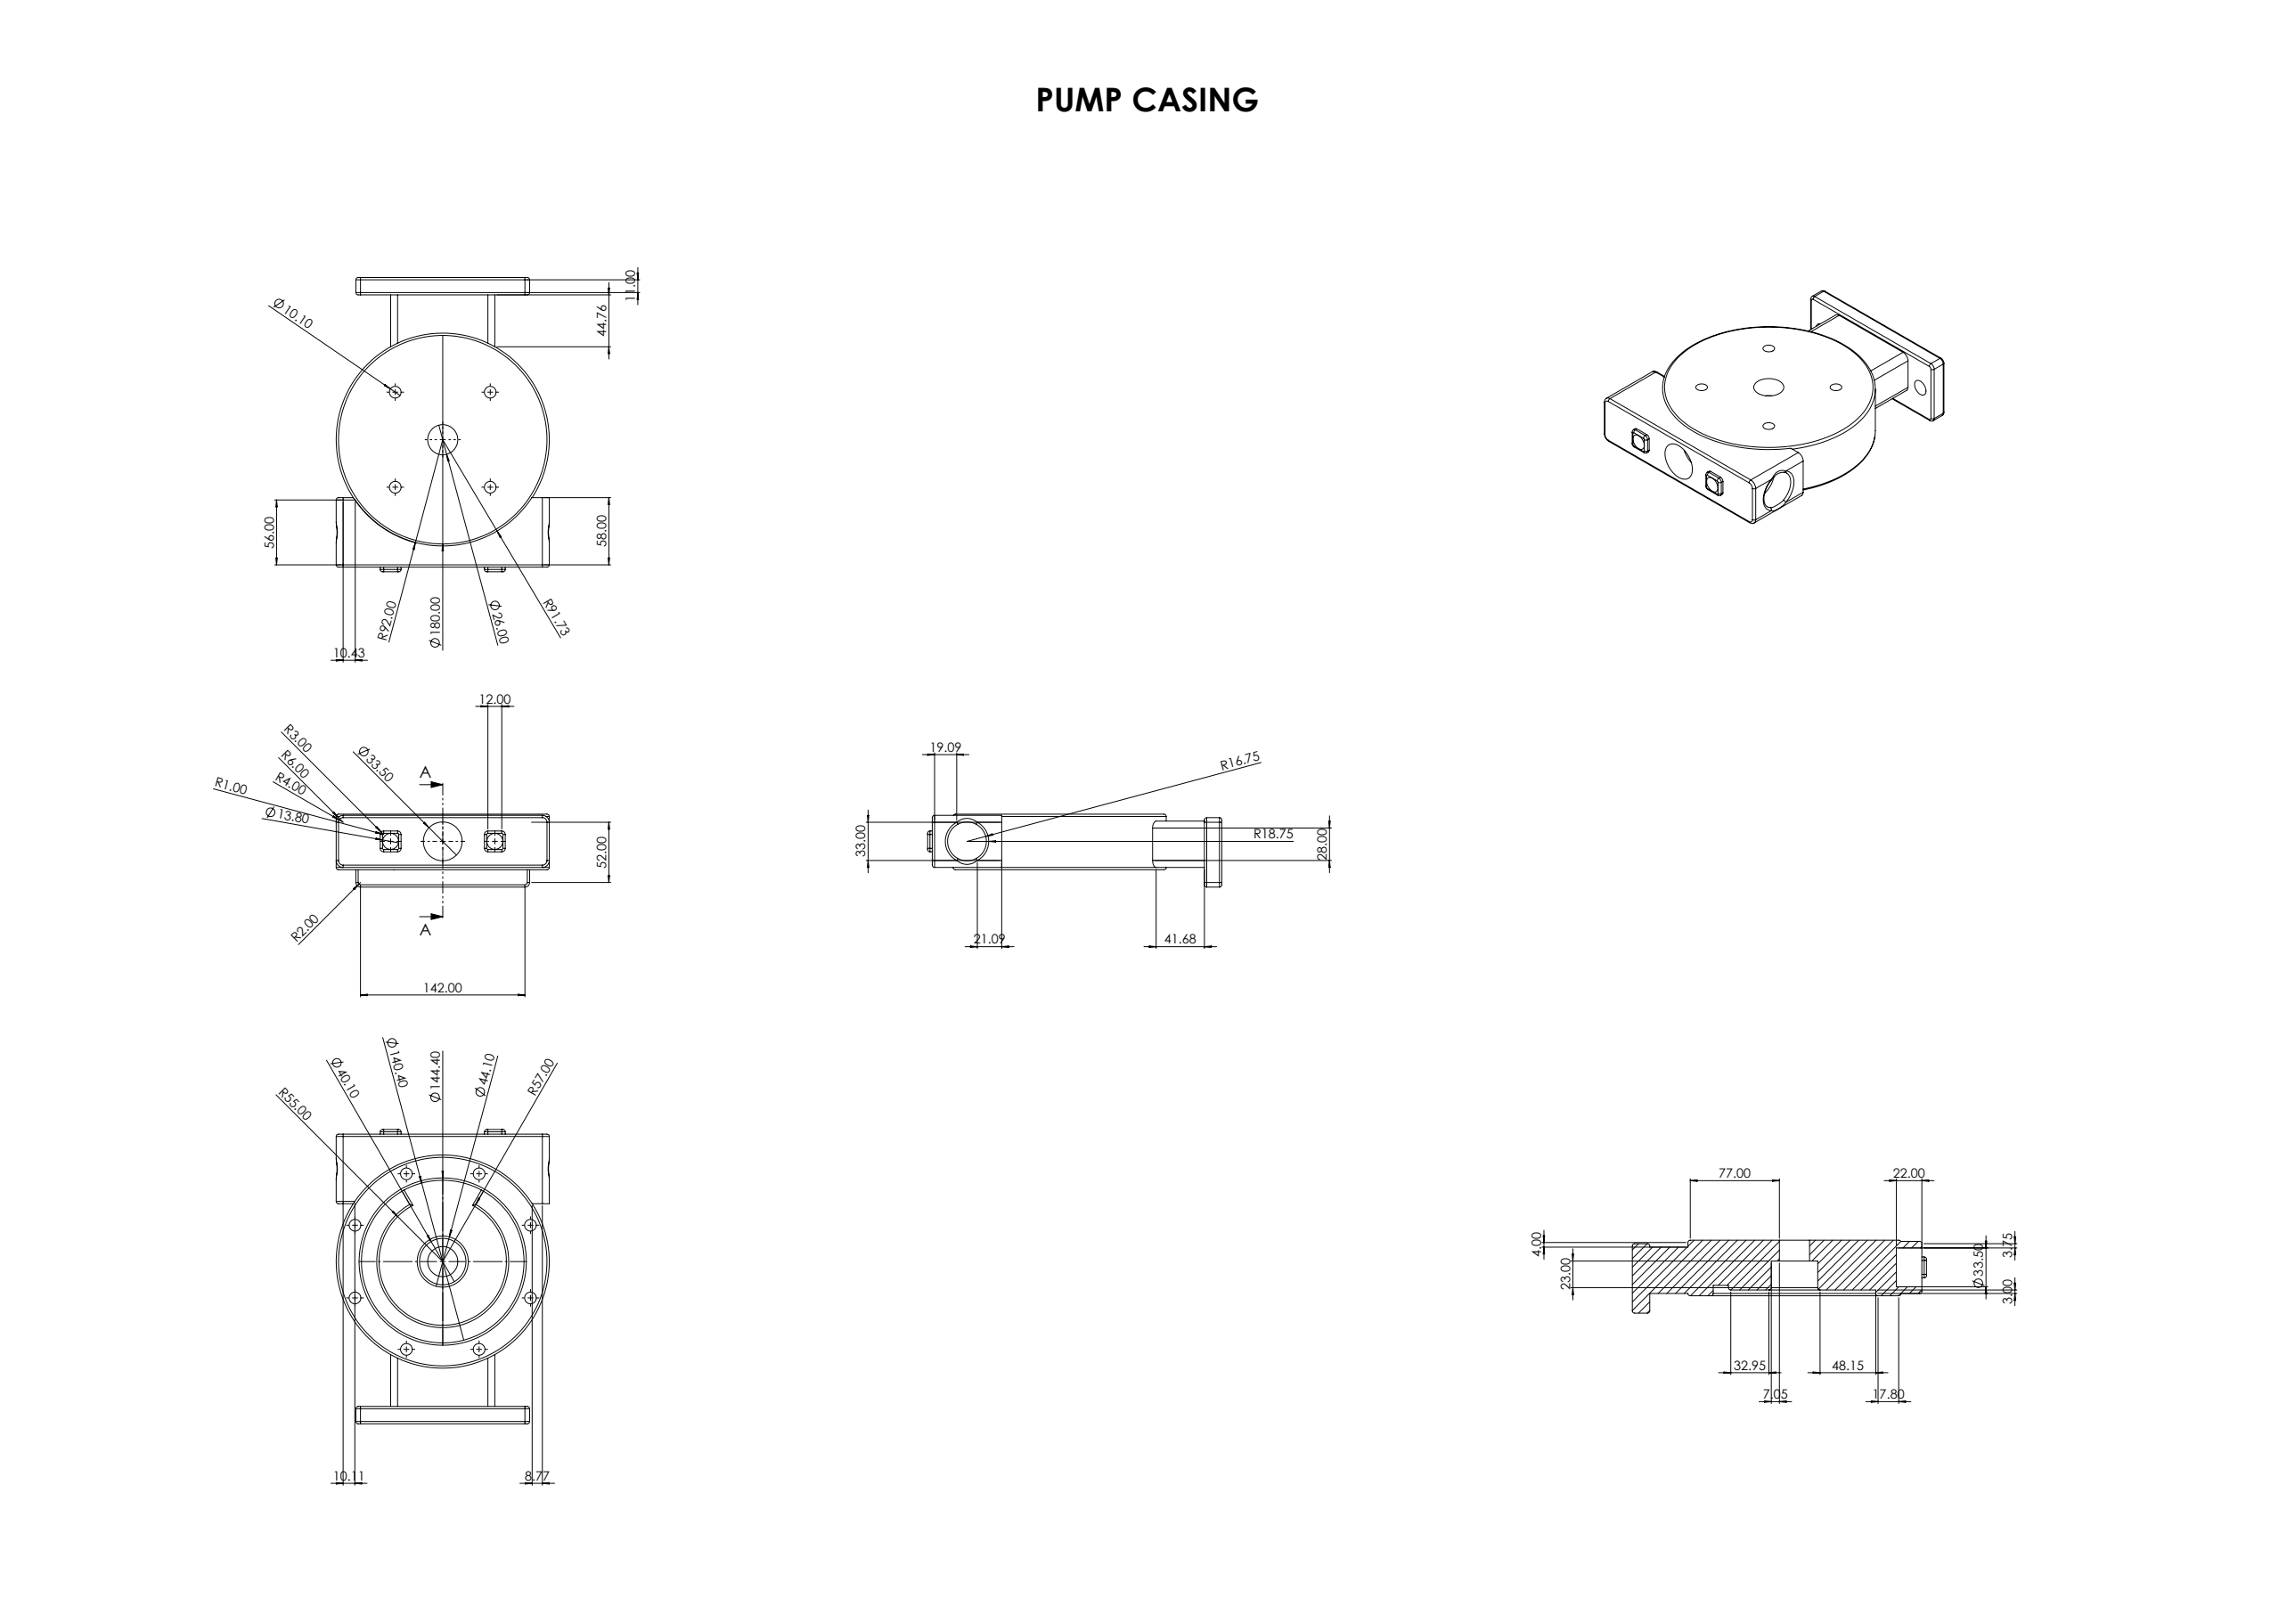
ISO-10303-21;
HEADER;
/* Generated by software containing ST-Developer
 * from STEP Tools, Inc. (www.steptools.com) 
 */

FILE_DESCRIPTION(
/* description */ (''),
/* implementation_level */ '2;1');

FILE_NAME(
/* name */ '01_Pump_Casing.step',
/* time_stamp */ '2026-10-26T04:15:57-07:00',
/* author */ (''),
/* organization */ (''),
/* preprocessor_version */ 'ST-DEVELOPER v20.2',
/* originating_system */ 'Autodesk Translation Framework v15.15.0.0',
/* authorisation */ '');

FILE_SCHEMA (('AUTOMOTIVE_DESIGN { 1 0 10303 214 3 1 1 }'));
ENDSEC;

DATA;
#10=MECHANICAL_DESIGN_GEOMETRIC_PRESENTATION_REPRESENTATION('',(#452),#55737);
#412=SHAPE_REPRESENTATION_RELATIONSHIP('SRR','None',#55821,#432);
#432=ADVANCED_BREP_SHAPE_REPRESENTATION('',(#472),#55717);
#452=STYLED_ITEM('',(#56005),#472);
#472=MANIFOLD_SOLID_BREP('Body1',#27221);
#492=B_SPLINE_SURFACE_WITH_KNOTS('',3,3,((#38041,#38042,#38043,#38044,#38045,
#38046,#38047,#38048),(#38049,#38050,#38051,#38052,#38053,#38054,#38055,
#38056),(#38057,#38058,#38059,#38060,#38061,#38062,#38063,#38064),(#38065,
#38066,#38067,#38068,#38069,#38070,#38071,#38072),(#38073,#38074,#38075,
#38076,#38077,#38078,#38079,#38080),(#38081,#38082,#38083,#38084,#38085,
#38086,#38087,#38088)),.UNSPECIFIED.,.F.,.F.,.F.,(4,1,1,4),(4,1,1,1,1,4),
(0.,0.285714285714286,0.571428571428571,1.),(0.,0.532095912060411,0.798143868090616,
1.06419182412082,1.59628773618123,1.86233569221144),.UNSPECIFIED.);
#493=B_SPLINE_SURFACE_WITH_KNOTS('',3,3,((#38114,#38115,#38116,#38117,#38118,
#38119,#38120,#38121),(#38122,#38123,#38124,#38125,#38126,#38127,#38128,
#38129),(#38130,#38131,#38132,#38133,#38134,#38135,#38136,#38137),(#38138,
#38139,#38140,#38141,#38142,#38143,#38144,#38145),(#38146,#38147,#38148,
#38149,#38150,#38151,#38152,#38153),(#38154,#38155,#38156,#38157,#38158,
#38159,#38160,#38161)),.UNSPECIFIED.,.F.,.F.,.F.,(4,1,1,4),(4,1,1,1,1,4),
(0.,0.285714285714286,0.571428571428571,1.),(8.87358627225765E-17,0.532095912059373,
0.798143868089059,1.06419182411875,1.33023978014843,1.8623356922078),
 .UNSPECIFIED.);
#494=B_SPLINE_SURFACE_WITH_KNOTS('',3,3,((#38313,#38314,#38315,#38316,#38317,
#38318,#38319,#38320,#38321),(#38322,#38323,#38324,#38325,#38326,#38327,
#38328,#38329,#38330),(#38331,#38332,#38333,#38334,#38335,#38336,#38337,
#38338,#38339),(#38340,#38341,#38342,#38343,#38344,#38345,#38346,#38347,
#38348),(#38349,#38350,#38351,#38352,#38353,#38354,#38355,#38356,#38357),
(#38358,#38359,#38360,#38361,#38362,#38363,#38364,#38365,#38366)),
 .UNSPECIFIED.,.F.,.F.,.F.,(4,1,1,4),(4,1,1,1,1,1,4),(0.,0.285714285714286,
0.571428571428571,1.),(0.,0.266047956030205,0.798143868090615,1.06419182412082,
1.33023978015103,1.46326375816613,1.86233569221144),.UNSPECIFIED.);
#495=B_SPLINE_SURFACE_WITH_KNOTS('',3,3,((#38384,#38385,#38386,#38387,#38388,
#38389,#38390,#38391),(#38392,#38393,#38394,#38395,#38396,#38397,#38398,
#38399),(#38400,#38401,#38402,#38403,#38404,#38405,#38406,#38407),(#38408,
#38409,#38410,#38411,#38412,#38413,#38414,#38415),(#38416,#38417,#38418,
#38419,#38420,#38421,#38422,#38423),(#38424,#38425,#38426,#38427,#38428,
#38429,#38430,#38431)),.UNSPECIFIED.,.F.,.F.,.F.,(4,1,1,4),(4,1,1,1,1,4),
(0.,0.285714285714286,0.571428571428571,1.),(2.59005157847017E-16,0.532095912059373,
0.79814386808906,1.06419182411875,1.59628773617812,1.86233569220781),
 .UNSPECIFIED.);
#584=(
BOUNDED_SURFACE()
B_SPLINE_SURFACE(2,2,((#37536,#37537,#37538),(#37539,#37540,#37541),(#37542,
#37543,#37544)),.UNSPECIFIED.,.F.,.F.,.F.)
B_SPLINE_SURFACE_WITH_KNOTS((3,3),(3,3),(-1.5707963267949,0.),(-3.14159265358979,
-1.5707963267949),.UNSPECIFIED.)
GEOMETRIC_REPRESENTATION_ITEM()
RATIONAL_B_SPLINE_SURFACE(((1.,0.707106781186549,1.),(0.707106781186545,
0.499999999999999,0.707106781186545),(1.,0.707106781186549,1.)))
REPRESENTATION_ITEM('')
SURFACE()
);
#585=(
BOUNDED_SURFACE()
B_SPLINE_SURFACE(2,2,((#37556,#37557,#37558),(#37559,#37560,#37561),(#37562,
#37563,#37564)),.UNSPECIFIED.,.F.,.F.,.F.)
B_SPLINE_SURFACE_WITH_KNOTS((3,3),(3,3),(-1.5707963267949,0.),(-1.5707963267949,
-4.44089209850058E-15),.UNSPECIFIED.)
GEOMETRIC_REPRESENTATION_ITEM()
RATIONAL_B_SPLINE_SURFACE(((1.,0.707106781186549,1.),(0.707106781186545,
0.499999999999999,0.707106781186545),(1.,0.707106781186549,1.)))
REPRESENTATION_ITEM('')
SURFACE()
);
#586=(
BOUNDED_SURFACE()
B_SPLINE_SURFACE(2,2,((#37576,#37577,#37578),(#37579,#37580,#37581),(#37582,
#37583,#37584)),.UNSPECIFIED.,.F.,.F.,.F.)
B_SPLINE_SURFACE_WITH_KNOTS((3,3),(3,3),(-1.5707963267949,0.),(4.4408920985006E-15,
1.57079632679489),.UNSPECIFIED.)
GEOMETRIC_REPRESENTATION_ITEM()
RATIONAL_B_SPLINE_SURFACE(((1.,0.70710678118655,1.),(0.707106781186545,
0.5,0.707106781186545),(1.,0.70710678118655,1.)))
REPRESENTATION_ITEM('')
SURFACE()
);
#587=(
BOUNDED_SURFACE()
B_SPLINE_SURFACE(2,2,((#37596,#37597,#37598),(#37599,#37600,#37601),(#37602,
#37603,#37604)),.UNSPECIFIED.,.F.,.F.,.F.)
B_SPLINE_SURFACE_WITH_KNOTS((3,3),(3,3),(-1.5707963267949,0.),(1.5707963267949,
3.14159265358979),.UNSPECIFIED.)
GEOMETRIC_REPRESENTATION_ITEM()
RATIONAL_B_SPLINE_SURFACE(((1.,0.707106781186549,1.),(0.707106781186545,
0.499999999999999,0.707106781186545),(1.,0.707106781186549,1.)))
REPRESENTATION_ITEM('')
SURFACE()
);
#588=(
BOUNDED_SURFACE()
B_SPLINE_SURFACE(2,2,((#37639,#37640,#37641),(#37642,#37643,#37644),(#37645,
#37646,#37647)),.UNSPECIFIED.,.F.,.F.,.F.)
B_SPLINE_SURFACE_WITH_KNOTS((3,3),(3,3),(0.,1.5707963267949),(-1.5707963267949,
-4.44089209850058E-15),.UNSPECIFIED.)
GEOMETRIC_REPRESENTATION_ITEM()
RATIONAL_B_SPLINE_SURFACE(((1.,0.707106781186549,1.),(0.707106781186545,
0.499999999999999,0.707106781186545),(1.,0.707106781186549,1.)))
REPRESENTATION_ITEM('')
SURFACE()
);
#589=(
BOUNDED_SURFACE()
B_SPLINE_SURFACE(2,2,((#37658,#37659,#37660),(#37661,#37662,#37663),(#37664,
#37665,#37666)),.UNSPECIFIED.,.F.,.F.,.F.)
B_SPLINE_SURFACE_WITH_KNOTS((3,3),(3,3),(0.,1.5707963267949),(4.4408920985006E-15,
1.57079632679489),.UNSPECIFIED.)
GEOMETRIC_REPRESENTATION_ITEM()
RATIONAL_B_SPLINE_SURFACE(((1.,0.70710678118655,1.),(0.707106781186545,
0.5,0.707106781186545),(1.,0.70710678118655,1.)))
REPRESENTATION_ITEM('')
SURFACE()
);
#590=(
BOUNDED_SURFACE()
B_SPLINE_SURFACE(2,2,((#37674,#37675,#37676),(#37677,#37678,#37679),(#37680,
#37681,#37682)),.UNSPECIFIED.,.F.,.F.,.F.)
B_SPLINE_SURFACE_WITH_KNOTS((3,3),(3,3),(0.,1.5707963267949),(1.5707963267949,
3.14159265358979),.UNSPECIFIED.)
GEOMETRIC_REPRESENTATION_ITEM()
RATIONAL_B_SPLINE_SURFACE(((1.,0.707106781186548,1.),(0.707106781186545,
0.499999999999999,0.707106781186545),(1.,0.707106781186548,1.)))
REPRESENTATION_ITEM('')
SURFACE()
);
#591=(
BOUNDED_SURFACE()
B_SPLINE_SURFACE(2,2,((#37690,#37691,#37692),(#37693,#37694,#37695),(#37696,
#37697,#37698)),.UNSPECIFIED.,.F.,.F.,.F.)
B_SPLINE_SURFACE_WITH_KNOTS((3,3),(3,3),(0.,1.5707963267949),(-3.14159265358979,
-1.5707963267949),.UNSPECIFIED.)
GEOMETRIC_REPRESENTATION_ITEM()
RATIONAL_B_SPLINE_SURFACE(((1.,0.70710678118655,1.),(0.707106781186545,
0.5,0.707106781186545),(1.,0.70710678118655,1.)))
REPRESENTATION_ITEM('')
SURFACE()
);
#592=(
BOUNDED_SURFACE()
B_SPLINE_SURFACE(2,2,((#37737,#37738,#37739),(#37740,#37741,#37742),(#37743,
#37744,#37745)),.UNSPECIFIED.,.F.,.F.,.F.)
B_SPLINE_SURFACE_WITH_KNOTS((3,3),(3,3),(0.,1.5707963267949),(-3.14159265358979,
-1.5707963267949),.UNSPECIFIED.)
GEOMETRIC_REPRESENTATION_ITEM()
RATIONAL_B_SPLINE_SURFACE(((1.,0.707106781186548,1.),(0.707106781186545,
0.499999999999999,0.707106781186545),(1.,0.707106781186548,1.)))
REPRESENTATION_ITEM('')
SURFACE()
);
#593=(
BOUNDED_SURFACE()
B_SPLINE_SURFACE(2,2,((#37757,#37758,#37759),(#37760,#37761,#37762),(#37763,
#37764,#37765)),.UNSPECIFIED.,.F.,.F.,.F.)
B_SPLINE_SURFACE_WITH_KNOTS((3,3),(3,3),(0.,1.5707963267949),(-1.5707963267949,
1.5832964389939E-15),.UNSPECIFIED.)
GEOMETRIC_REPRESENTATION_ITEM()
RATIONAL_B_SPLINE_SURFACE(((1.,0.707106781186545,1.),(0.707106781186551,
0.500000000000001,0.707106781186551),(1.,0.707106781186545,1.)))
REPRESENTATION_ITEM('')
SURFACE()
);
#594=(
BOUNDED_SURFACE()
B_SPLINE_SURFACE(2,2,((#37777,#37778,#37779),(#37780,#37781,#37782),(#37783,
#37784,#37785)),.UNSPECIFIED.,.F.,.F.,.F.)
B_SPLINE_SURFACE_WITH_KNOTS((3,3),(3,3),(0.,1.5707963267949),(-1.3322676295502E-14,
1.5707963267949),.UNSPECIFIED.)
GEOMETRIC_REPRESENTATION_ITEM()
RATIONAL_B_SPLINE_SURFACE(((1.,0.707106781186541,1.),(0.707106781186549,
0.499999999999996,0.707106781186549),(1.,0.707106781186541,1.)))
REPRESENTATION_ITEM('')
SURFACE()
);
#595=(
BOUNDED_SURFACE()
B_SPLINE_SURFACE(2,2,((#37797,#37798,#37799),(#37800,#37801,#37802),(#37803,
#37804,#37805)),.UNSPECIFIED.,.F.,.F.,.F.)
B_SPLINE_SURFACE_WITH_KNOTS((3,3),(3,3),(0.,1.5707963267949),(1.5707963267949,
3.1415926535898),.UNSPECIFIED.)
GEOMETRIC_REPRESENTATION_ITEM()
RATIONAL_B_SPLINE_SURFACE(((1.,0.707106781186546,1.),(0.707106781186545,
0.499999999999997,0.707106781186545),(1.,0.707106781186546,1.)))
REPRESENTATION_ITEM('')
SURFACE()
);
#596=(
BOUNDED_SURFACE()
B_SPLINE_SURFACE(2,2,((#37838,#37839,#37840),(#37841,#37842,#37843),(#37844,
#37845,#37846)),.UNSPECIFIED.,.F.,.F.,.F.)
B_SPLINE_SURFACE_WITH_KNOTS((3,3),(3,3),(0.,1.5707963267949),(-3.14159265358979,
-1.57079632679489),.UNSPECIFIED.)
GEOMETRIC_REPRESENTATION_ITEM()
RATIONAL_B_SPLINE_SURFACE(((1.,0.707106781186547,1.),(0.707106781186556,
0.500000000000006,0.707106781186556),(1.,0.707106781186547,1.)))
REPRESENTATION_ITEM('')
SURFACE()
);
#597=(
BOUNDED_SURFACE()
B_SPLINE_SURFACE(2,2,((#37858,#37859,#37860),(#37861,#37862,#37863),(#37864,
#37865,#37866)),.UNSPECIFIED.,.F.,.F.,.F.)
B_SPLINE_SURFACE_WITH_KNOTS((3,3),(3,3),(0.,1.5707963267949),(-1.5707963267949,
0.),.UNSPECIFIED.)
GEOMETRIC_REPRESENTATION_ITEM()
RATIONAL_B_SPLINE_SURFACE(((1.,0.707106781186548,1.),(0.707106781186545,
0.499999999999998,0.707106781186545),(1.,0.707106781186548,1.)))
REPRESENTATION_ITEM('')
SURFACE()
);
#598=(
BOUNDED_SURFACE()
B_SPLINE_SURFACE(2,2,((#37878,#37879,#37880),(#37881,#37882,#37883),(#37884,
#37885,#37886)),.UNSPECIFIED.,.F.,.F.,.F.)
B_SPLINE_SURFACE_WITH_KNOTS((3,3),(3,3),(0.,1.5707963267949),(-4.4408920985006E-15,
1.5707963267949),.UNSPECIFIED.)
GEOMETRIC_REPRESENTATION_ITEM()
RATIONAL_B_SPLINE_SURFACE(((1.,0.707106781186546,1.),(0.707106781186545,
0.499999999999997,0.707106781186545),(1.,0.707106781186546,1.)))
REPRESENTATION_ITEM('')
SURFACE()
);
#599=(
BOUNDED_SURFACE()
B_SPLINE_SURFACE(2,2,((#37898,#37899,#37900),(#37901,#37902,#37903),(#37904,
#37905,#37906)),.UNSPECIFIED.,.F.,.F.,.F.)
B_SPLINE_SURFACE_WITH_KNOTS((3,3),(3,3),(0.,1.5707963267949),(1.57079632679489,
3.14159265358981),.UNSPECIFIED.)
GEOMETRIC_REPRESENTATION_ITEM()
RATIONAL_B_SPLINE_SURFACE(((1.,0.70710678118654,1.),(0.707106781186558,
0.500000000000002,0.707106781186558),(1.,0.70710678118654,1.)))
REPRESENTATION_ITEM('')
SURFACE()
);
#605=FACE_BOUND('',#8400,.T.);
#606=FACE_BOUND('',#8401,.T.);
#607=FACE_BOUND('',#8402,.T.);
#608=FACE_BOUND('',#8403,.T.);
#609=FACE_BOUND('',#8404,.T.);
#610=FACE_BOUND('',#8407,.T.);
#611=FACE_BOUND('',#8408,.T.);
#612=FACE_BOUND('',#8409,.T.);
#613=FACE_BOUND('',#8410,.T.);
#614=FACE_BOUND('',#8411,.T.);
#615=FACE_BOUND('',#8412,.T.);
#616=FACE_BOUND('',#8413,.T.);
#617=FACE_BOUND('',#8414,.T.);
#618=FACE_BOUND('',#8415,.T.);
#619=FACE_BOUND('',#8429,.T.);
#620=FACE_BOUND('',#8430,.T.);
#621=FACE_BOUND('',#8443,.T.);
#622=FACE_BOUND('',#8444,.T.);
#623=FACE_BOUND('',#8445,.T.);
#624=FACE_BOUND('',#8459,.T.);
#625=FACE_BOUND('',#8473,.T.);
#626=FACE_BOUND('',#8478,.T.);
#627=FACE_BOUND('',#8511,.T.);
#628=FACE_BOUND('',#8512,.T.);
#629=FACE_BOUND('',#8513,.T.);
#630=FACE_BOUND('',#8558,.T.);
#757=PLANE('',#27475);
#758=PLANE('',#27486);
#759=PLANE('',#27518);
#760=PLANE('',#27521);
#761=PLANE('',#27522);
#762=PLANE('',#27543);
#763=PLANE('',#27545);
#764=PLANE('',#27546);
#765=PLANE('',#27575);
#766=PLANE('',#27578);
#767=PLANE('',#27579);
#768=PLANE('',#27603);
#769=PLANE('',#27606);
#770=PLANE('',#27607);
#771=PLANE('',#27620);
#772=PLANE('',#27628);
#773=PLANE('',#27631);
#774=PLANE('',#27646);
#775=PLANE('',#27664);
#776=PLANE('',#27665);
#777=PLANE('',#27688);
#778=PLANE('',#27690);
#779=PLANE('',#27713);
#780=PLANE('',#27716);
#781=PLANE('',#27719);
#782=PLANE('',#27720);
#783=PLANE('',#27721);
#784=PLANE('',#27722);
#785=PLANE('',#27723);
#786=PLANE('',#27726);
#787=PLANE('',#27729);
#788=PLANE('',#27732);
#789=PLANE('',#27735);
#790=PLANE('',#27738);
#791=PLANE('',#27741);
#792=PLANE('',#27744);
#793=PLANE('',#27747);
#794=PLANE('',#27750);
#795=PLANE('',#27753);
#796=PLANE('',#27756);
#797=PLANE('',#27759);
#798=PLANE('',#27760);
#799=PLANE('',#27761);
#800=PLANE('',#27765);
#801=PLANE('',#27767);
#802=PLANE('',#27769);
#803=PLANE('',#27771);
#804=PLANE('',#27774);
#805=PLANE('',#27776);
#806=PLANE('',#27778);
#807=PLANE('',#27780);
#808=PLANE('',#27781);
#809=PLANE('',#27783);
#1758=LINE('',#37415,#4129);
#1759=LINE('',#37432,#4130);
#1760=LINE('',#37458,#4131);
#1761=LINE('',#37484,#4132);
#1762=LINE('',#37532,#4133);
#1763=LINE('',#37535,#4134);
#1764=LINE('',#37554,#4135);
#1765=LINE('',#37555,#4136);
#1766=LINE('',#37574,#4137);
#1767=LINE('',#37575,#4138);
#1768=LINE('',#37594,#4139);
#1769=LINE('',#37595,#4140);
#1770=LINE('',#37609,#4141);
#1771=LINE('',#37612,#4142);
#1772=LINE('',#37615,#4143);
#1773=LINE('',#37616,#4144);
#1774=LINE('',#37619,#4145);
#1775=LINE('',#37623,#4146);
#1776=LINE('',#37624,#4147);
#1777=LINE('',#37635,#4148);
#1778=LINE('',#37638,#4149);
#1779=LINE('',#37656,#4150);
#1780=LINE('',#37657,#4151);
#1781=LINE('',#37673,#4152);
#1782=LINE('',#37689,#4153);
#1783=LINE('',#37702,#4154);
#1784=LINE('',#37704,#4155);
#1785=LINE('',#37706,#4156);
#1786=LINE('',#37712,#4157);
#1787=LINE('',#37716,#4158);
#1788=LINE('',#37720,#4159);
#1789=LINE('',#37723,#4160);
#1790=LINE('',#37733,#4161);
#1791=LINE('',#37736,#4162);
#1792=LINE('',#37755,#4163);
#1793=LINE('',#37756,#4164);
#1794=LINE('',#37775,#4165);
#1795=LINE('',#37776,#4166);
#1796=LINE('',#37795,#4167);
#1797=LINE('',#37796,#4168);
#1798=LINE('',#37810,#4169);
#1799=LINE('',#37813,#4170);
#1800=LINE('',#37816,#4171);
#1801=LINE('',#37817,#4172);
#1802=LINE('',#37820,#4173);
#1803=LINE('',#37824,#4174);
#1804=LINE('',#37825,#4175);
#1805=LINE('',#37834,#4176);
#1806=LINE('',#37837,#4177);
#1807=LINE('',#37856,#4178);
#1808=LINE('',#37857,#4179);
#1809=LINE('',#37876,#4180);
#1810=LINE('',#37877,#4181);
#1811=LINE('',#37896,#4182);
#1812=LINE('',#37897,#4183);
#1813=LINE('',#37911,#4184);
#1814=LINE('',#37914,#4185);
#1815=LINE('',#37917,#4186);
#1816=LINE('',#37918,#4187);
#1817=LINE('',#37921,#4188);
#1818=LINE('',#37925,#4189);
#1819=LINE('',#37926,#4190);
#1820=LINE('',#37936,#4191);
#1821=LINE('',#37940,#4192);
#1822=LINE('',#37966,#4193);
#1823=LINE('',#37976,#4194);
#1824=LINE('',#37978,#4195);
#1825=LINE('',#37982,#4196);
#1826=LINE('',#37986,#4197);
#1827=LINE('',#38019,#4198);
#1828=LINE('',#38022,#4199);
#1829=LINE('',#38023,#4200);
#1830=LINE('',#38026,#4201);
#1831=LINE('',#38029,#4202);
#1832=LINE('',#38180,#4203);
#1833=LINE('',#38184,#4204);
#1834=LINE('',#38187,#4205);
#1835=LINE('',#38190,#4206);
#1836=LINE('',#38191,#4207);
#1837=LINE('',#38194,#4208);
#1838=LINE('',#38198,#4209);
#1839=LINE('',#38201,#4210);
#1840=LINE('',#38207,#4211);
#1841=LINE('',#38210,#4212);
#1842=LINE('',#38218,#4213);
#1843=LINE('',#38219,#4214);
#1844=LINE('',#38225,#4215);
#1845=LINE('',#38229,#4216);
#1846=LINE('',#38240,#4217);
#1847=LINE('',#38242,#4218);
#1848=LINE('',#38243,#4219);
#1849=LINE('',#38249,#4220);
#1850=LINE('',#38252,#4221);
#1851=LINE('',#38260,#4222);
#1852=LINE('',#38268,#4223);
#1853=LINE('',#38279,#4224);
#1854=LINE('',#38280,#4225);
#1855=LINE('',#38286,#4226);
#1856=LINE('',#38292,#4227);
#1857=LINE('',#38295,#4228);
#1858=LINE('',#38299,#4229);
#1859=LINE('',#38302,#4230);
#1860=LINE('',#38449,#4231);
#1861=LINE('',#38450,#4232);
#1862=LINE('',#38453,#4233);
#1863=LINE('',#38456,#4234);
#1864=LINE('',#38458,#4235);
#1865=LINE('',#38461,#4236);
#1866=LINE('',#38466,#4237);
#1867=LINE('',#38471,#4238);
#1868=LINE('',#38479,#4239);
#1869=LINE('',#38480,#4240);
#1870=LINE('',#38483,#4241);
#1871=LINE('',#38488,#4242);
#1872=LINE('',#38493,#4243);
#1873=LINE('',#38498,#4244);
#1874=LINE('',#38503,#4245);
#1875=LINE('',#38508,#4246);
#1876=LINE('',#38513,#4247);
#1877=LINE('',#38518,#4248);
#1878=LINE('',#38523,#4249);
#1879=LINE('',#38528,#4250);
#1880=LINE('',#38533,#4251);
#1881=LINE('',#38538,#4252);
#1882=LINE('',#38546,#4253);
#1883=LINE('',#38548,#4254);
#1884=LINE('',#38550,#4255);
#1885=LINE('',#38552,#4256);
#1886=LINE('',#38555,#4257);
#1887=LINE('',#38557,#4258);
#1888=LINE('',#38559,#4259);
#1889=LINE('',#38563,#4260);
#1890=LINE('',#38564,#4261);
#1891=LINE('',#38566,#4262);
#1892=LINE('',#38568,#4263);
#1893=LINE('',#38570,#4264);
#1894=LINE('',#38572,#4265);
#1895=LINE('',#38574,#4266);
#1896=LINE('',#38576,#4267);
#1897=LINE('',#38580,#4268);
#1898=LINE('',#38583,#4269);
#4129=VECTOR('',#29994,10.);
#4130=VECTOR('',#29999,10.);
#4131=VECTOR('',#30002,10.);
#4132=VECTOR('',#30005,10.);
#4133=VECTOR('',#30052,10.);
#4134=VECTOR('',#30055,10.);
#4135=VECTOR('',#30066,10.);
#4136=VECTOR('',#30067,10.);
#4137=VECTOR('',#30078,10.);
#4138=VECTOR('',#30079,10.);
#4139=VECTOR('',#30090,10.);
#4140=VECTOR('',#30091,10.);
#4141=VECTOR('',#30098,10.);
#4142=VECTOR('',#30101,10.);
#4143=VECTOR('',#30104,10.);
#4144=VECTOR('',#30105,10.);
#4145=VECTOR('',#30108,10.);
#4146=VECTOR('',#30113,10.);
#4147=VECTOR('',#30114,10.);
#4148=VECTOR('',#30125,10.);
#4149=VECTOR('',#30128,10.);
#4150=VECTOR('',#30139,10.);
#4151=VECTOR('',#30140,10.);
#4152=VECTOR('',#30149,10.);
#4153=VECTOR('',#30158,10.);
#4154=VECTOR('',#30165,10.);
#4155=VECTOR('',#30168,10.);
#4156=VECTOR('',#30171,10.);
#4157=VECTOR('',#30176,10.);
#4158=VECTOR('',#30179,10.);
#4159=VECTOR('',#30182,10.);
#4160=VECTOR('',#30185,10.);
#4161=VECTOR('',#30194,10.);
#4162=VECTOR('',#30197,10.);
#4163=VECTOR('',#30208,10.);
#4164=VECTOR('',#30209,10.);
#4165=VECTOR('',#30220,10.);
#4166=VECTOR('',#30221,10.);
#4167=VECTOR('',#30232,10.);
#4168=VECTOR('',#30233,10.);
#4169=VECTOR('',#30240,10.);
#4170=VECTOR('',#30243,10.);
#4171=VECTOR('',#30246,10.);
#4172=VECTOR('',#30247,10.);
#4173=VECTOR('',#30250,10.);
#4174=VECTOR('',#30255,10.);
#4175=VECTOR('',#30256,10.);
#4176=VECTOR('',#30265,10.);
#4177=VECTOR('',#30268,10.);
#4178=VECTOR('',#30279,10.);
#4179=VECTOR('',#30280,10.);
#4180=VECTOR('',#30291,10.);
#4181=VECTOR('',#30292,10.);
#4182=VECTOR('',#30303,10.);
#4183=VECTOR('',#30304,10.);
#4184=VECTOR('',#30311,10.);
#4185=VECTOR('',#30314,10.);
#4186=VECTOR('',#30317,10.);
#4187=VECTOR('',#30318,10.);
#4188=VECTOR('',#30321,10.);
#4189=VECTOR('',#30326,10.);
#4190=VECTOR('',#30327,10.);
#4191=VECTOR('',#30340,70.2);
#4192=VECTOR('',#30343,10.);
#4193=VECTOR('',#30346,10.);
#4194=VECTOR('',#30359,10.);
#4195=VECTOR('',#30360,10.);
#4196=VECTOR('',#30365,20.05);
#4197=VECTOR('',#30370,10.);
#4198=VECTOR('',#30377,10.);
#4199=VECTOR('',#30380,10.);
#4200=VECTOR('',#30381,10.);
#4201=VECTOR('',#30384,10.);
#4202=VECTOR('',#30389,10.);
#4203=VECTOR('',#30414,10.);
#4204=VECTOR('',#30417,10.);
#4205=VECTOR('',#30420,10.);
#4206=VECTOR('',#30423,10.);
#4207=VECTOR('',#30424,10.);
#4208=VECTOR('',#30427,16.75);
#4209=VECTOR('',#30432,10.);
#4210=VECTOR('',#30435,10.);
#4211=VECTOR('',#30440,10.);
#4212=VECTOR('',#30443,10.);
#4213=VECTOR('',#30454,10.);
#4214=VECTOR('',#30455,10.);
#4215=VECTOR('',#30464,10.);
#4216=VECTOR('',#30467,10.);
#4217=VECTOR('',#30468,10.);
#4218=VECTOR('',#30471,10.);
#4219=VECTOR('',#30472,10.);
#4220=VECTOR('',#30479,10.);
#4221=VECTOR('',#30482,10.);
#4222=VECTOR('',#30493,10.);
#4223=VECTOR('',#30504,10.);
#4224=VECTOR('',#30517,10.);
#4225=VECTOR('',#30518,10.);
#4226=VECTOR('',#30527,10.);
#4227=VECTOR('',#30534,10.);
#4228=VECTOR('',#30537,10.);
#4229=VECTOR('',#30540,10.);
#4230=VECTOR('',#30543,10.);
#4231=VECTOR('',#30568,10.);
#4232=VECTOR('',#30569,10.);
#4233=VECTOR('',#30572,16.75);
#4234=VECTOR('',#30577,7.);
#4235=VECTOR('',#30580,7.);
#4236=VECTOR('',#30583,6.9);
#4237=VECTOR('',#30590,6.9);
#4238=VECTOR('',#30597,16.75);
#4239=VECTOR('',#30610,10.);
#4240=VECTOR('',#30611,10.);
#4241=VECTOR('',#30614,5.05);
#4242=VECTOR('',#30621,5.05);
#4243=VECTOR('',#30628,5.05);
#4244=VECTOR('',#30635,5.05);
#4245=VECTOR('',#30642,5.05);
#4246=VECTOR('',#30649,5.05);
#4247=VECTOR('',#30656,5.05);
#4248=VECTOR('',#30663,5.05);
#4249=VECTOR('',#30670,5.05);
#4250=VECTOR('',#30677,5.05);
#4251=VECTOR('',#30684,5.05);
#4252=VECTOR('',#30691,5.05);
#4253=VECTOR('',#30704,13.);
#4254=VECTOR('',#30707,10.);
#4255=VECTOR('',#30710,10.);
#4256=VECTOR('',#30713,10.);
#4257=VECTOR('',#30718,10.);
#4258=VECTOR('',#30721,10.);
#4259=VECTOR('',#30724,10.);
#4260=VECTOR('',#30731,10.);
#4261=VECTOR('',#30732,10.);
#4262=VECTOR('',#30735,10.);
#4263=VECTOR('',#30738,10.);
#4264=VECTOR('',#30741,10.);
#4265=VECTOR('',#30744,10.);
#4266=VECTOR('',#30747,10.);
#4267=VECTOR('',#30750,10.);
#4268=VECTOR('',#30755,10.);
#4269=VECTOR('',#30760,10.);
#6500=CYLINDRICAL_SURFACE('',#27470,92.);
#6501=CYLINDRICAL_SURFACE('',#27496,2.);
#6502=CYLINDRICAL_SURFACE('',#27502,2.);
#6503=CYLINDRICAL_SURFACE('',#27507,2.);
#6504=CYLINDRICAL_SURFACE('',#27512,2.);
#6505=CYLINDRICAL_SURFACE('',#27516,4.00000000000002);
#6506=CYLINDRICAL_SURFACE('',#27519,4.00000000000002);
#6507=CYLINDRICAL_SURFACE('',#27525,2.);
#6508=CYLINDRICAL_SURFACE('',#27531,2.);
#6509=CYLINDRICAL_SURFACE('',#27535,2.);
#6510=CYLINDRICAL_SURFACE('',#27539,2.);
#6511=CYLINDRICAL_SURFACE('',#27544,4.00000000000002);
#6512=CYLINDRICAL_SURFACE('',#27553,2.);
#6513=CYLINDRICAL_SURFACE('',#27559,2.);
#6514=CYLINDRICAL_SURFACE('',#27564,2.);
#6515=CYLINDRICAL_SURFACE('',#27569,2.);
#6516=CYLINDRICAL_SURFACE('',#27573,3.);
#6517=CYLINDRICAL_SURFACE('',#27576,3.00000000000001);
#6518=CYLINDRICAL_SURFACE('',#27581,2.);
#6519=CYLINDRICAL_SURFACE('',#27587,2.);
#6520=CYLINDRICAL_SURFACE('',#27592,2.);
#6521=CYLINDRICAL_SURFACE('',#27597,2.);
#6522=CYLINDRICAL_SURFACE('',#27601,3.);
#6523=CYLINDRICAL_SURFACE('',#27604,2.99999999999999);
#6524=CYLINDRICAL_SURFACE('',#27612,70.2);
#6525=CYLINDRICAL_SURFACE('',#27622,20.05);
#6526=CYLINDRICAL_SURFACE('',#27624,2.);
#6527=CYLINDRICAL_SURFACE('',#27627,2.);
#6528=CYLINDRICAL_SURFACE('',#27629,57.);
#6529=CYLINDRICAL_SURFACE('',#27643,5.99999999999997);
#6530=CYLINDRICAL_SURFACE('',#27647,16.75);
#6531=CYLINDRICAL_SURFACE('',#27649,2.);
#6532=CYLINDRICAL_SURFACE('',#27651,2.);
#6533=CYLINDRICAL_SURFACE('',#27658,2.);
#6534=CYLINDRICAL_SURFACE('',#27662,5.99999999999996);
#6535=CYLINDRICAL_SURFACE('',#27666,2.);
#6536=CYLINDRICAL_SURFACE('',#27672,2.);
#6537=CYLINDRICAL_SURFACE('',#27677,2.);
#6538=CYLINDRICAL_SURFACE('',#27683,2.);
#6539=CYLINDRICAL_SURFACE('',#27706,5.99999999999999);
#6540=CYLINDRICAL_SURFACE('',#27707,16.75);
#6541=CYLINDRICAL_SURFACE('',#27709,7.);
#6542=CYLINDRICAL_SURFACE('',#27710,7.);
#6543=CYLINDRICAL_SURFACE('',#27711,6.9);
#6544=CYLINDRICAL_SURFACE('',#27714,6.9);
#6545=CYLINDRICAL_SURFACE('',#27717,16.75);
#6546=CYLINDRICAL_SURFACE('',#27724,5.05);
#6547=CYLINDRICAL_SURFACE('',#27727,5.05);
#6548=CYLINDRICAL_SURFACE('',#27730,5.05);
#6549=CYLINDRICAL_SURFACE('',#27733,5.05);
#6550=CYLINDRICAL_SURFACE('',#27736,5.05);
#6551=CYLINDRICAL_SURFACE('',#27739,5.05);
#6552=CYLINDRICAL_SURFACE('',#27742,5.05);
#6553=CYLINDRICAL_SURFACE('',#27745,5.05);
#6554=CYLINDRICAL_SURFACE('',#27748,5.05);
#6555=CYLINDRICAL_SURFACE('',#27751,5.05);
#6556=CYLINDRICAL_SURFACE('',#27754,5.05);
#6557=CYLINDRICAL_SURFACE('',#27757,5.05);
#6558=CYLINDRICAL_SURFACE('',#27763,13.);
#6559=CYLINDRICAL_SURFACE('',#27764,2.99999999999999);
#6560=CYLINDRICAL_SURFACE('',#27766,3.00000000000001);
#6561=CYLINDRICAL_SURFACE('',#27768,3.);
#6562=CYLINDRICAL_SURFACE('',#27770,2.99999999999999);
#6563=CYLINDRICAL_SURFACE('',#27772,4.00000000000001);
#6564=CYLINDRICAL_SURFACE('',#27773,6.00000000000001);
#6565=CYLINDRICAL_SURFACE('',#27775,6.00000000000001);
#6566=CYLINDRICAL_SURFACE('',#27777,6.00000000000001);
#6567=CYLINDRICAL_SURFACE('',#27779,6.00000000000001);
#6568=CYLINDRICAL_SURFACE('',#27784,5.99999999999998);
#6827=FACE_OUTER_BOUND('',#8397,.T.);
#6828=FACE_OUTER_BOUND('',#8398,.T.);
#6829=FACE_OUTER_BOUND('',#8399,.T.);
#6830=FACE_OUTER_BOUND('',#8405,.T.);
#6831=FACE_OUTER_BOUND('',#8406,.T.);
#6832=FACE_OUTER_BOUND('',#8416,.T.);
#6833=FACE_OUTER_BOUND('',#8417,.T.);
#6834=FACE_OUTER_BOUND('',#8418,.T.);
#6835=FACE_OUTER_BOUND('',#8419,.T.);
#6836=FACE_OUTER_BOUND('',#8420,.T.);
#6837=FACE_OUTER_BOUND('',#8421,.T.);
#6838=FACE_OUTER_BOUND('',#8422,.T.);
#6839=FACE_OUTER_BOUND('',#8423,.T.);
#6840=FACE_OUTER_BOUND('',#8424,.T.);
#6841=FACE_OUTER_BOUND('',#8425,.T.);
#6842=FACE_OUTER_BOUND('',#8426,.T.);
#6843=FACE_OUTER_BOUND('',#8427,.T.);
#6844=FACE_OUTER_BOUND('',#8428,.T.);
#6845=FACE_OUTER_BOUND('',#8431,.T.);
#6846=FACE_OUTER_BOUND('',#8432,.T.);
#6847=FACE_OUTER_BOUND('',#8433,.T.);
#6848=FACE_OUTER_BOUND('',#8434,.T.);
#6849=FACE_OUTER_BOUND('',#8435,.T.);
#6850=FACE_OUTER_BOUND('',#8436,.T.);
#6851=FACE_OUTER_BOUND('',#8437,.T.);
#6852=FACE_OUTER_BOUND('',#8438,.T.);
#6853=FACE_OUTER_BOUND('',#8439,.T.);
#6854=FACE_OUTER_BOUND('',#8440,.T.);
#6855=FACE_OUTER_BOUND('',#8441,.T.);
#6856=FACE_OUTER_BOUND('',#8442,.T.);
#6857=FACE_OUTER_BOUND('',#8446,.T.);
#6858=FACE_OUTER_BOUND('',#8447,.T.);
#6859=FACE_OUTER_BOUND('',#8448,.T.);
#6860=FACE_OUTER_BOUND('',#8449,.T.);
#6861=FACE_OUTER_BOUND('',#8450,.T.);
#6862=FACE_OUTER_BOUND('',#8451,.T.);
#6863=FACE_OUTER_BOUND('',#8452,.T.);
#6864=FACE_OUTER_BOUND('',#8453,.T.);
#6865=FACE_OUTER_BOUND('',#8454,.T.);
#6866=FACE_OUTER_BOUND('',#8455,.T.);
#6867=FACE_OUTER_BOUND('',#8456,.T.);
#6868=FACE_OUTER_BOUND('',#8457,.T.);
#6869=FACE_OUTER_BOUND('',#8458,.T.);
#6870=FACE_OUTER_BOUND('',#8460,.T.);
#6871=FACE_OUTER_BOUND('',#8461,.T.);
#6872=FACE_OUTER_BOUND('',#8462,.T.);
#6873=FACE_OUTER_BOUND('',#8463,.T.);
#6874=FACE_OUTER_BOUND('',#8464,.T.);
#6875=FACE_OUTER_BOUND('',#8465,.T.);
#6876=FACE_OUTER_BOUND('',#8466,.T.);
#6877=FACE_OUTER_BOUND('',#8467,.T.);
#6878=FACE_OUTER_BOUND('',#8468,.T.);
#6879=FACE_OUTER_BOUND('',#8469,.T.);
#6880=FACE_OUTER_BOUND('',#8470,.T.);
#6881=FACE_OUTER_BOUND('',#8471,.T.);
#6882=FACE_OUTER_BOUND('',#8472,.T.);
#6883=FACE_OUTER_BOUND('',#8474,.T.);
#6884=FACE_OUTER_BOUND('',#8475,.T.);
#6885=FACE_OUTER_BOUND('',#8476,.T.);
#6886=FACE_OUTER_BOUND('',#8477,.T.);
#6887=FACE_OUTER_BOUND('',#8479,.T.);
#6888=FACE_OUTER_BOUND('',#8480,.T.);
#6889=FACE_OUTER_BOUND('',#8481,.T.);
#6890=FACE_OUTER_BOUND('',#8482,.T.);
#6891=FACE_OUTER_BOUND('',#8483,.T.);
#6892=FACE_OUTER_BOUND('',#8484,.T.);
#6893=FACE_OUTER_BOUND('',#8485,.T.);
#6894=FACE_OUTER_BOUND('',#8486,.T.);
#6895=FACE_OUTER_BOUND('',#8487,.T.);
#6896=FACE_OUTER_BOUND('',#8488,.T.);
#6897=FACE_OUTER_BOUND('',#8489,.T.);
#6898=FACE_OUTER_BOUND('',#8490,.T.);
#6899=FACE_OUTER_BOUND('',#8491,.T.);
#6900=FACE_OUTER_BOUND('',#8492,.T.);
#6901=FACE_OUTER_BOUND('',#8493,.T.);
#6902=FACE_OUTER_BOUND('',#8494,.T.);
#6903=FACE_OUTER_BOUND('',#8495,.T.);
#6904=FACE_OUTER_BOUND('',#8496,.T.);
#6905=FACE_OUTER_BOUND('',#8497,.T.);
#6906=FACE_OUTER_BOUND('',#8498,.T.);
#6907=FACE_OUTER_BOUND('',#8499,.T.);
#6908=FACE_OUTER_BOUND('',#8500,.T.);
#6909=FACE_OUTER_BOUND('',#8501,.T.);
#6910=FACE_OUTER_BOUND('',#8502,.T.);
#6911=FACE_OUTER_BOUND('',#8503,.T.);
#6912=FACE_OUTER_BOUND('',#8504,.T.);
#6913=FACE_OUTER_BOUND('',#8505,.T.);
#6914=FACE_OUTER_BOUND('',#8506,.T.);
#6915=FACE_OUTER_BOUND('',#8507,.T.);
#6916=FACE_OUTER_BOUND('',#8508,.T.);
#6917=FACE_OUTER_BOUND('',#8509,.T.);
#6918=FACE_OUTER_BOUND('',#8510,.T.);
#6919=FACE_OUTER_BOUND('',#8514,.T.);
#6920=FACE_OUTER_BOUND('',#8515,.T.);
#6921=FACE_OUTER_BOUND('',#8516,.T.);
#6922=FACE_OUTER_BOUND('',#8517,.T.);
#6923=FACE_OUTER_BOUND('',#8518,.T.);
#6924=FACE_OUTER_BOUND('',#8519,.T.);
#6925=FACE_OUTER_BOUND('',#8520,.T.);
#6926=FACE_OUTER_BOUND('',#8521,.T.);
#6927=FACE_OUTER_BOUND('',#8522,.T.);
#6928=FACE_OUTER_BOUND('',#8523,.T.);
#6929=FACE_OUTER_BOUND('',#8524,.T.);
#6930=FACE_OUTER_BOUND('',#8525,.T.);
#6931=FACE_OUTER_BOUND('',#8526,.T.);
#6932=FACE_OUTER_BOUND('',#8527,.T.);
#6933=FACE_OUTER_BOUND('',#8528,.T.);
#6934=FACE_OUTER_BOUND('',#8529,.T.);
#6935=FACE_OUTER_BOUND('',#8530,.T.);
#6936=FACE_OUTER_BOUND('',#8531,.T.);
#6937=FACE_OUTER_BOUND('',#8532,.T.);
#6938=FACE_OUTER_BOUND('',#8533,.T.);
#6939=FACE_OUTER_BOUND('',#8534,.T.);
#6940=FACE_OUTER_BOUND('',#8535,.T.);
#6941=FACE_OUTER_BOUND('',#8536,.T.);
#6942=FACE_OUTER_BOUND('',#8537,.T.);
#6943=FACE_OUTER_BOUND('',#8538,.T.);
#6944=FACE_OUTER_BOUND('',#8539,.T.);
#6945=FACE_OUTER_BOUND('',#8540,.T.);
#6946=FACE_OUTER_BOUND('',#8541,.T.);
#6947=FACE_OUTER_BOUND('',#8542,.T.);
#6948=FACE_OUTER_BOUND('',#8543,.T.);
#6949=FACE_OUTER_BOUND('',#8544,.T.);
#6950=FACE_OUTER_BOUND('',#8545,.T.);
#6951=FACE_OUTER_BOUND('',#8546,.T.);
#6952=FACE_OUTER_BOUND('',#8547,.T.);
#6953=FACE_OUTER_BOUND('',#8548,.T.);
#6954=FACE_OUTER_BOUND('',#8549,.T.);
#6955=FACE_OUTER_BOUND('',#8550,.T.);
#6956=FACE_OUTER_BOUND('',#8551,.T.);
#6957=FACE_OUTER_BOUND('',#8552,.T.);
#6958=FACE_OUTER_BOUND('',#8553,.T.);
#6959=FACE_OUTER_BOUND('',#8554,.T.);
#6960=FACE_OUTER_BOUND('',#8555,.T.);
#6961=FACE_OUTER_BOUND('',#8556,.T.);
#6962=FACE_OUTER_BOUND('',#8557,.T.);
#6963=FACE_OUTER_BOUND('',#8559,.T.);
#6964=FACE_OUTER_BOUND('',#8560,.T.);
#6965=FACE_OUTER_BOUND('',#8561,.T.);
#6966=FACE_OUTER_BOUND('',#8562,.T.);
#6967=FACE_OUTER_BOUND('',#8563,.T.);
#6968=FACE_OUTER_BOUND('',#8564,.T.);
#6969=FACE_OUTER_BOUND('',#8565,.T.);
#6970=FACE_OUTER_BOUND('',#8566,.T.);
#6971=FACE_OUTER_BOUND('',#8567,.T.);
#6972=FACE_OUTER_BOUND('',#8568,.T.);
#6973=FACE_OUTER_BOUND('',#8569,.T.);
#6974=FACE_OUTER_BOUND('',#8570,.T.);
#6975=FACE_OUTER_BOUND('',#8571,.T.);
#6976=FACE_OUTER_BOUND('',#8572,.T.);
#6977=FACE_OUTER_BOUND('',#8573,.T.);
#6978=FACE_OUTER_BOUND('',#8574,.T.);
#6979=FACE_OUTER_BOUND('',#8575,.T.);
#6980=FACE_OUTER_BOUND('',#8576,.T.);
#6981=FACE_OUTER_BOUND('',#8577,.T.);
#6982=FACE_OUTER_BOUND('',#8578,.T.);
#6983=FACE_OUTER_BOUND('',#8579,.T.);
#8397=EDGE_LOOP('',(#17802,#17803,#17804,#17805,#17806,#17807,#17808,#17809));
#8398=EDGE_LOOP('',(#17810,#17811,#17812,#17813,#17814,#17815,#17816,#17817,
#17818,#17819,#17820,#17821,#17822,#17823,#17824,#17825));
#8399=EDGE_LOOP('',(#17826));
#8400=EDGE_LOOP('',(#17827));
#8401=EDGE_LOOP('',(#17828));
#8402=EDGE_LOOP('',(#17829));
#8403=EDGE_LOOP('',(#17830));
#8404=EDGE_LOOP('',(#17831));
#8405=EDGE_LOOP('',(#17832,#17833,#17834,#17835,#17836,#17837,#17838,#17839));
#8406=EDGE_LOOP('',(#17840));
#8407=EDGE_LOOP('',(#17841));
#8408=EDGE_LOOP('',(#17842));
#8409=EDGE_LOOP('',(#17843));
#8410=EDGE_LOOP('',(#17844));
#8411=EDGE_LOOP('',(#17845));
#8412=EDGE_LOOP('',(#17846));
#8413=EDGE_LOOP('',(#17847));
#8414=EDGE_LOOP('',(#17848));
#8415=EDGE_LOOP('',(#17849));
#8416=EDGE_LOOP('',(#17850,#17851,#17852,#17853));
#8417=EDGE_LOOP('',(#17854,#17855,#17856,#17857));
#8418=EDGE_LOOP('',(#17858,#17859,#17860,#17861));
#8419=EDGE_LOOP('',(#17862,#17863,#17864,#17865));
#8420=EDGE_LOOP('',(#17866,#17867,#17868,#17869));
#8421=EDGE_LOOP('',(#17870,#17871,#17872,#17873));
#8422=EDGE_LOOP('',(#17874,#17875,#17876,#17877));
#8423=EDGE_LOOP('',(#17878,#17879,#17880,#17881));
#8424=EDGE_LOOP('',(#17882,#17883,#17884,#17885));
#8425=EDGE_LOOP('',(#17886,#17887,#17888,#17889));
#8426=EDGE_LOOP('',(#17890,#17891,#17892,#17893));
#8427=EDGE_LOOP('',(#17894,#17895,#17896,#17897));
#8428=EDGE_LOOP('',(#17898,#17899,#17900,#17901,#17902,#17903,#17904,#17905));
#8429=EDGE_LOOP('',(#17906));
#8430=EDGE_LOOP('',(#17907));
#8431=EDGE_LOOP('',(#17908,#17909,#17910,#17911));
#8432=EDGE_LOOP('',(#17912,#17913,#17914,#17915));
#8433=EDGE_LOOP('',(#17916,#17917,#17918,#17919));
#8434=EDGE_LOOP('',(#17920,#17921,#17922,#17923));
#8435=EDGE_LOOP('',(#17924,#17925,#17926,#17927));
#8436=EDGE_LOOP('',(#17928,#17929,#17930,#17931));
#8437=EDGE_LOOP('',(#17932,#17933,#17934,#17935));
#8438=EDGE_LOOP('',(#17936,#17937,#17938,#17939));
#8439=EDGE_LOOP('',(#17940,#17941,#17942,#17943));
#8440=EDGE_LOOP('',(#17944,#17945,#17946,#17947));
#8441=EDGE_LOOP('',(#17948,#17949,#17950,#17951));
#8442=EDGE_LOOP('',(#17952,#17953,#17954,#17955,#17956,#17957,#17958,#17959));
#8443=EDGE_LOOP('',(#17960,#17961,#17962,#17963,#17964,#17965,#17966,#17967));
#8444=EDGE_LOOP('',(#17968));
#8445=EDGE_LOOP('',(#17969));
#8446=EDGE_LOOP('',(#17970,#17971,#17972,#17973));
#8447=EDGE_LOOP('',(#17974,#17975,#17976,#17977));
#8448=EDGE_LOOP('',(#17978,#17979,#17980,#17981));
#8449=EDGE_LOOP('',(#17982,#17983,#17984,#17985));
#8450=EDGE_LOOP('',(#17986,#17987,#17988,#17989));
#8451=EDGE_LOOP('',(#17990,#17991,#17992,#17993));
#8452=EDGE_LOOP('',(#17994,#17995,#17996,#17997));
#8453=EDGE_LOOP('',(#17998,#17999,#18000,#18001));
#8454=EDGE_LOOP('',(#18002,#18003,#18004,#18005));
#8455=EDGE_LOOP('',(#18006,#18007,#18008,#18009));
#8456=EDGE_LOOP('',(#18010,#18011,#18012,#18013));
#8457=EDGE_LOOP('',(#18014,#18015,#18016,#18017));
#8458=EDGE_LOOP('',(#18018,#18019,#18020,#18021,#18022,#18023,#18024,#18025));
#8459=EDGE_LOOP('',(#18026));
#8460=EDGE_LOOP('',(#18027,#18028,#18029,#18030));
#8461=EDGE_LOOP('',(#18031,#18032,#18033,#18034));
#8462=EDGE_LOOP('',(#18035,#18036,#18037,#18038));
#8463=EDGE_LOOP('',(#18039,#18040,#18041,#18042));
#8464=EDGE_LOOP('',(#18043,#18044,#18045,#18046));
#8465=EDGE_LOOP('',(#18047,#18048,#18049,#18050));
#8466=EDGE_LOOP('',(#18051,#18052,#18053,#18054));
#8467=EDGE_LOOP('',(#18055,#18056,#18057,#18058));
#8468=EDGE_LOOP('',(#18059,#18060,#18061,#18062));
#8469=EDGE_LOOP('',(#18063,#18064,#18065,#18066));
#8470=EDGE_LOOP('',(#18067,#18068,#18069,#18070));
#8471=EDGE_LOOP('',(#18071,#18072,#18073,#18074));
#8472=EDGE_LOOP('',(#18075,#18076,#18077,#18078,#18079,#18080,#18081,#18082));
#8473=EDGE_LOOP('',(#18083));
#8474=EDGE_LOOP('',(#18084,#18085,#18086,#18087));
#8475=EDGE_LOOP('',(#18088,#18089,#18090,#18091,#18092,#18093,#18094,#18095,
#18096,#18097));
#8476=EDGE_LOOP('',(#18098,#18099,#18100,#18101));
#8477=EDGE_LOOP('',(#18102,#18103,#18104,#18105));
#8478=EDGE_LOOP('',(#18106));
#8479=EDGE_LOOP('',(#18107,#18108,#18109,#18110));
#8480=EDGE_LOOP('',(#18111,#18112,#18113,#18114));
#8481=EDGE_LOOP('',(#18115,#18116,#18117,#18118));
#8482=EDGE_LOOP('',(#18119,#18120,#18121,#18122));
#8483=EDGE_LOOP('',(#18123,#18124,#18125,#18126));
#8484=EDGE_LOOP('',(#18127,#18128,#18129,#18130));
#8485=EDGE_LOOP('',(#18131,#18132,#18133,#18134));
#8486=EDGE_LOOP('',(#18135,#18136,#18137,#18138,#18139));
#8487=EDGE_LOOP('',(#18140,#18141,#18142,#18143));
#8488=EDGE_LOOP('',(#18144,#18145,#18146,#18147));
#8489=EDGE_LOOP('',(#18148,#18149,#18150,#18151));
#8490=EDGE_LOOP('',(#18152,#18153,#18154,#18155,#18156,#18157));
#8491=EDGE_LOOP('',(#18158,#18159,#18160,#18161));
#8492=EDGE_LOOP('',(#18162,#18163,#18164,#18165,#18166,#18167,#18168,#18169));
#8493=EDGE_LOOP('',(#18170,#18171,#18172,#18173,#18174));
#8494=EDGE_LOOP('',(#18175,#18176,#18177,#18178));
#8495=EDGE_LOOP('',(#18179,#18180,#18181,#18182));
#8496=EDGE_LOOP('',(#18183,#18184,#18185,#18186));
#8497=EDGE_LOOP('',(#18187,#18188,#18189,#18190));
#8498=EDGE_LOOP('',(#18191,#18192,#18193,#18194,#18195,#18196));
#8499=EDGE_LOOP('',(#18197,#18198,#18199,#18200,#18201,#18202));
#8500=EDGE_LOOP('',(#18203,#18204,#18205,#18206,#18207,#18208));
#8501=EDGE_LOOP('',(#18209,#18210,#18211,#18212));
#8502=EDGE_LOOP('',(#18213,#18214,#18215,#18216));
#8503=EDGE_LOOP('',(#18217,#18218,#18219,#18220));
#8504=EDGE_LOOP('',(#18221,#18222,#18223,#18224));
#8505=EDGE_LOOP('',(#18225,#18226,#18227,#18228));
#8506=EDGE_LOOP('',(#18229,#18230,#18231,#18232));
#8507=EDGE_LOOP('',(#18233,#18234,#18235,#18236));
#8508=EDGE_LOOP('',(#18237,#18238,#18239,#18240));
#8509=EDGE_LOOP('',(#18241,#18242,#18243,#18244));
#8510=EDGE_LOOP('',(#18245,#18246,#18247,#18248,#18249,#18250,#18251,#18252));
#8511=EDGE_LOOP('',(#18253,#18254,#18255,#18256,#18257,#18258,#18259,#18260));
#8512=EDGE_LOOP('',(#18261,#18262,#18263,#18264,#18265,#18266,#18267,#18268));
#8513=EDGE_LOOP('',(#18269));
#8514=EDGE_LOOP('',(#18270,#18271,#18272,#18273,#18274));
#8515=EDGE_LOOP('',(#18275,#18276,#18277,#18278));
#8516=EDGE_LOOP('',(#18279,#18280,#18281,#18282));
#8517=EDGE_LOOP('',(#18283,#18284,#18285,#18286));
#8518=EDGE_LOOP('',(#18287,#18288,#18289,#18290,#18291,#18292));
#8519=EDGE_LOOP('',(#18293,#18294,#18295,#18296,#18297,#18298,#18299,#18300));
#8520=EDGE_LOOP('',(#18301,#18302,#18303,#18304));
#8521=EDGE_LOOP('',(#18305,#18306,#18307,#18308));
#8522=EDGE_LOOP('',(#18309,#18310,#18311,#18312));
#8523=EDGE_LOOP('',(#18313));
#8524=EDGE_LOOP('',(#18314,#18315,#18316,#18317));
#8525=EDGE_LOOP('',(#18318));
#8526=EDGE_LOOP('',(#18319,#18320,#18321,#18322));
#8527=EDGE_LOOP('',(#18323));
#8528=EDGE_LOOP('',(#18324));
#8529=EDGE_LOOP('',(#18325,#18326,#18327,#18328));
#8530=EDGE_LOOP('',(#18329));
#8531=EDGE_LOOP('',(#18330,#18331,#18332,#18333));
#8532=EDGE_LOOP('',(#18334,#18335,#18336,#18337));
#8533=EDGE_LOOP('',(#18338));
#8534=EDGE_LOOP('',(#18339,#18340,#18341,#18342));
#8535=EDGE_LOOP('',(#18343));
#8536=EDGE_LOOP('',(#18344,#18345,#18346,#18347));
#8537=EDGE_LOOP('',(#18348));
#8538=EDGE_LOOP('',(#18349,#18350,#18351,#18352));
#8539=EDGE_LOOP('',(#18353));
#8540=EDGE_LOOP('',(#18354,#18355,#18356,#18357));
#8541=EDGE_LOOP('',(#18358));
#8542=EDGE_LOOP('',(#18359,#18360,#18361,#18362));
#8543=EDGE_LOOP('',(#18363));
#8544=EDGE_LOOP('',(#18364,#18365,#18366,#18367));
#8545=EDGE_LOOP('',(#18368));
#8546=EDGE_LOOP('',(#18369,#18370,#18371,#18372));
#8547=EDGE_LOOP('',(#18373));
#8548=EDGE_LOOP('',(#18374,#18375,#18376,#18377));
#8549=EDGE_LOOP('',(#18378));
#8550=EDGE_LOOP('',(#18379,#18380,#18381,#18382));
#8551=EDGE_LOOP('',(#18383));
#8552=EDGE_LOOP('',(#18384,#18385,#18386,#18387));
#8553=EDGE_LOOP('',(#18388));
#8554=EDGE_LOOP('',(#18389,#18390,#18391,#18392));
#8555=EDGE_LOOP('',(#18393));
#8556=EDGE_LOOP('',(#18394,#18395,#18396,#18397,#18398));
#8557=EDGE_LOOP('',(#18399));
#8558=EDGE_LOOP('',(#18400));
#8559=EDGE_LOOP('',(#18401,#18402,#18403,#18404));
#8560=EDGE_LOOP('',(#18405,#18406,#18407,#18408));
#8561=EDGE_LOOP('',(#18409,#18410,#18411,#18412));
#8562=EDGE_LOOP('',(#18413,#18414,#18415,#18416));
#8563=EDGE_LOOP('',(#18417,#18418,#18419,#18420));
#8564=EDGE_LOOP('',(#18421,#18422,#18423,#18424));
#8565=EDGE_LOOP('',(#18425,#18426,#18427,#18428));
#8566=EDGE_LOOP('',(#18429,#18430,#18431,#18432));
#8567=EDGE_LOOP('',(#18433,#18434,#18435,#18436));
#8568=EDGE_LOOP('',(#18437,#18438,#18439,#18440));
#8569=EDGE_LOOP('',(#18441,#18442,#18443,#18444));
#8570=EDGE_LOOP('',(#18445,#18446,#18447,#18448));
#8571=EDGE_LOOP('',(#18449,#18450,#18451,#18452));
#8572=EDGE_LOOP('',(#18453,#18454,#18455,#18456));
#8573=EDGE_LOOP('',(#18457,#18458,#18459,#18460));
#8574=EDGE_LOOP('',(#18461,#18462,#18463,#18464));
#8575=EDGE_LOOP('',(#18465,#18466,#18467,#18468));
#8576=EDGE_LOOP('',(#18469,#18470,#18471,#18472));
#8577=EDGE_LOOP('',(#18473,#18474,#18475,#18476,#18477,#18478,#18479));
#8578=EDGE_LOOP('',(#18480,#18481,#18482,#18483,#18484,#18485));
#8579=EDGE_LOOP('',(#18486,#18487,#18488,#18489,#18490,#18491));
#10119=CIRCLE('',#27465,92.);
#10120=CIRCLE('',#27466,2.);
#10121=CIRCLE('',#27467,90.);
#10122=CIRCLE('',#27468,92.);
#10123=CIRCLE('',#27469,91.7320508075689);
#10124=CIRCLE('',#27471,92.);
#10125=CIRCLE('',#27472,92.);
#10126=CIRCLE('',#27473,92.);
#10127=CIRCLE('',#27474,92.);
#10128=CIRCLE('',#27476,5.05);
#10129=CIRCLE('',#27477,5.05);
#10130=CIRCLE('',#27478,5.05);
#10131=CIRCLE('',#27479,5.05);
#10132=CIRCLE('',#27480,13.);
#10133=CIRCLE('',#27482,2.);
#10134=CIRCLE('',#27483,90.);
#10135=CIRCLE('',#27484,92.);
#10136=CIRCLE('',#27485,92.);
#10137=CIRCLE('',#27487,5.05);
#10138=CIRCLE('',#27488,5.05);
#10139=CIRCLE('',#27489,5.05);
#10140=CIRCLE('',#27490,5.05);
#10141=CIRCLE('',#27491,5.05);
#10142=CIRCLE('',#27492,5.05);
#10143=CIRCLE('',#27493,5.05);
#10144=CIRCLE('',#27494,5.05);
#10145=CIRCLE('',#27495,72.2);
#10146=CIRCLE('',#27497,2.);
#10147=CIRCLE('',#27498,1.99999999999999);
#10148=CIRCLE('',#27499,1.99999999999999);
#10149=CIRCLE('',#27500,4.00000000000001);
#10150=CIRCLE('',#27501,2.00000000000001);
#10151=CIRCLE('',#27503,1.99999999999999);
#10152=CIRCLE('',#27504,1.99999999999999);
#10153=CIRCLE('',#27505,4.00000000000002);
#10154=CIRCLE('',#27506,2.00000000000002);
#10155=CIRCLE('',#27508,1.99999999999999);
#10156=CIRCLE('',#27509,1.99999999999999);
#10157=CIRCLE('',#27510,4.00000000000002);
#10158=CIRCLE('',#27511,2.00000000000002);
#10159=CIRCLE('',#27513,1.99999999999999);
#10160=CIRCLE('',#27514,4.00000000000002);
#10161=CIRCLE('',#27515,2.00000000000002);
#10162=CIRCLE('',#27517,4.00000000000002);
#10163=CIRCLE('',#27520,4.00000000000002);
#10164=CIRCLE('',#27523,7.);
#10165=CIRCLE('',#27524,7.);
#10166=CIRCLE('',#27526,1.99999999999999);
#10167=CIRCLE('',#27527,2.);
#10168=CIRCLE('',#27528,1.99999999999999);
#10169=CIRCLE('',#27529,2.00000000000002);
#10170=CIRCLE('',#27530,4.00000000000002);
#10171=CIRCLE('',#27532,2.);
#10172=CIRCLE('',#27533,2.);
#10173=CIRCLE('',#27534,2.00000000000002);
#10174=CIRCLE('',#27536,2.);
#10175=CIRCLE('',#27537,2.);
#10176=CIRCLE('',#27538,2.00000000000002);
#10177=CIRCLE('',#27540,2.);
#10178=CIRCLE('',#27541,2.00000000000001);
#10179=CIRCLE('',#27542,4.00000000000001);
#10180=CIRCLE('',#27547,6.00000000000001);
#10181=CIRCLE('',#27548,6.00000000000001);
#10182=CIRCLE('',#27549,6.00000000000001);
#10183=CIRCLE('',#27550,6.00000000000001);
#10184=CIRCLE('',#27551,7.);
#10185=CIRCLE('',#27552,7.);
#10186=CIRCLE('',#27554,1.99999999999998);
#10187=CIRCLE('',#27555,2.);
#10188=CIRCLE('',#27556,2.);
#10189=CIRCLE('',#27557,1.00000000000001);
#10190=CIRCLE('',#27558,3.00000000000001);
#10191=CIRCLE('',#27560,2.);
#10192=CIRCLE('',#27561,2.);
#10193=CIRCLE('',#27562,0.999999999999996);
#10194=CIRCLE('',#27563,3.);
#10195=CIRCLE('',#27565,2.);
#10196=CIRCLE('',#27566,2.);
#10197=CIRCLE('',#27567,0.999999999999989);
#10198=CIRCLE('',#27568,2.99999999999999);
#10199=CIRCLE('',#27570,2.);
#10200=CIRCLE('',#27571,0.999999999999998);
#10201=CIRCLE('',#27572,3.);
#10202=CIRCLE('',#27574,3.);
#10203=CIRCLE('',#27577,3.00000000000001);
#10204=CIRCLE('',#27580,6.9);
#10205=CIRCLE('',#27582,1.99999999999998);
#10206=CIRCLE('',#27583,2.);
#10207=CIRCLE('',#27584,2.);
#10208=CIRCLE('',#27585,0.999999999999993);
#10209=CIRCLE('',#27586,2.99999999999999);
#10210=CIRCLE('',#27588,2.);
#10211=CIRCLE('',#27589,2.);
#10212=CIRCLE('',#27590,1.);
#10213=CIRCLE('',#27591,3.);
#10214=CIRCLE('',#27593,2.);
#10215=CIRCLE('',#27594,2.);
#10216=CIRCLE('',#27595,1.00000000000001);
#10217=CIRCLE('',#27596,3.00000000000001);
#10218=CIRCLE('',#27598,2.);
#10219=CIRCLE('',#27599,0.999999999999989);
#10220=CIRCLE('',#27600,2.99999999999999);
#10221=CIRCLE('',#27602,3.);
#10222=CIRCLE('',#27605,2.99999999999999);
#10223=CIRCLE('',#27608,6.9);
#10224=CIRCLE('',#27610,2.);
#10225=CIRCLE('',#27611,70.2);
#10226=CIRCLE('',#27613,70.2);
#10227=CIRCLE('',#27614,70.2);
#10228=CIRCLE('',#27615,70.2);
#10229=CIRCLE('',#27617,22.05);
#10230=CIRCLE('',#27618,2.);
#10231=CIRCLE('',#27619,20.05);
#10232=CIRCLE('',#27621,55.);
#10233=CIRCLE('',#27623,20.05);
#10234=CIRCLE('',#27626,57.);
#10235=CIRCLE('',#27630,57.);
#10236=CIRCLE('',#27633,2.00000000000001);
#10237=CIRCLE('',#27634,16.75);
#10238=CIRCLE('',#27635,16.75);
#10239=CIRCLE('',#27636,1.99999999999999);
#10240=CIRCLE('',#27637,18.75);
#10241=CIRCLE('',#27638,2.);
#10242=CIRCLE('',#27640,2.);
#10243=CIRCLE('',#27641,18.75);
#10244=CIRCLE('',#27642,16.75);
#10245=CIRCLE('',#27644,5.99999999999997);
#10246=CIRCLE('',#27645,5.99999999999997);
#10247=CIRCLE('',#27648,16.75);
#10248=CIRCLE('',#27650,2.);
#10249=CIRCLE('',#27652,1.99999999999999);
#10250=CIRCLE('',#27653,2.);
#10251=CIRCLE('',#27655,2.);
#10252=CIRCLE('',#27656,5.99999999999996);
#10253=CIRCLE('',#27657,3.99999999999996);
#10254=CIRCLE('',#27660,5.99999999999999);
#10255=CIRCLE('',#27661,3.99999999999999);
#10256=CIRCLE('',#27663,5.99999999999996);
#10257=CIRCLE('',#27667,1.99999999999999);
#10258=CIRCLE('',#27668,1.99999999999999);
#10259=CIRCLE('',#27670,2.);
#10260=CIRCLE('',#27671,3.99999999999996);
#10261=CIRCLE('',#27673,2.);
#10262=CIRCLE('',#27675,2.00000000000001);
#10263=CIRCLE('',#27676,3.99999999999997);
#10264=CIRCLE('',#27678,1.99999999999999);
#10265=CIRCLE('',#27680,2.);
#10266=CIRCLE('',#27681,3.99999999999998);
#10267=CIRCLE('',#27682,5.99999999999998);
#10268=CIRCLE('',#27684,2.);
#10269=CIRCLE('',#27686,3.99999999999999);
#10270=CIRCLE('',#27687,5.99999999999999);
#10271=CIRCLE('',#27689,18.75);
#10272=CIRCLE('',#27691,3.);
#10273=CIRCLE('',#27692,2.99999999999999);
#10274=CIRCLE('',#27693,2.99999999999999);
#10275=CIRCLE('',#27694,3.00000000000001);
#10276=CIRCLE('',#27695,16.75);
#10277=CIRCLE('',#27697,1.99999999999999);
#10278=CIRCLE('',#27698,16.75);
#10279=CIRCLE('',#27699,16.75);
#10280=CIRCLE('',#27700,2.00000000000001);
#10281=CIRCLE('',#27701,2.);
#10282=CIRCLE('',#27703,1.99999999999999);
#10283=CIRCLE('',#27704,18.75);
#10284=CIRCLE('',#27705,16.75);
#10285=CIRCLE('',#27708,16.75);
#10286=CIRCLE('',#27712,6.9);
#10287=CIRCLE('',#27715,6.9);
#10288=CIRCLE('',#27718,16.75);
#10289=CIRCLE('',#27725,5.05);
#10290=CIRCLE('',#27728,5.05);
#10291=CIRCLE('',#27731,5.05);
#10292=CIRCLE('',#27734,5.05);
#10293=CIRCLE('',#27737,5.05);
#10294=CIRCLE('',#27740,5.05);
#10295=CIRCLE('',#27743,5.05);
#10296=CIRCLE('',#27746,5.05);
#10297=CIRCLE('',#27749,5.05);
#10298=CIRCLE('',#27752,5.05);
#10299=CIRCLE('',#27755,5.05);
#10300=CIRCLE('',#27758,5.05);
#10301=CIRCLE('',#27762,13.);
#10302=CIRCLE('',#27782,5.99999999999998);
#10978=B_SPLINE_CURVE_WITH_KNOTS('',3,(#37380,#37381,#37382,#37383,#37384,
#37385),.UNSPECIFIED.,.F.,.F.,(4,2,4),(0.,0.0698759495705014,0.100813530301716),
 .UNSPECIFIED.);
#10979=B_SPLINE_CURVE_WITH_KNOTS('',3,(#37394,#37395,#37396,#37397,#37398,
#37399,#37400,#37401,#37402,#37403,#37404,#37405,#37406,#37407,#37408,#37409,
#37410,#37411),.UNSPECIFIED.,.F.,.F.,(4,2,2,2,2,2,2,2,4),(0.229981338184207,
0.230186209246776,0.230825449288754,0.23191142362845,0.236130991491961,
0.265789540903692,0.330613311085503,0.427893531851159,0.499880951546163),
 .UNSPECIFIED.);
#10980=B_SPLINE_CURVE_WITH_KNOTS('',3,(#37421,#37422,#37423,#37424,#37425,
#37426,#37427,#37428,#37429,#37430),.UNSPECIFIED.,.F.,.F.,(4,2,2,2,4),(-0.959890977249723,
-0.705434126471362,-0.450977275693002,-0.225488637846501,0.),
 .UNSPECIFIED.);
#10981=B_SPLINE_CURVE_WITH_KNOTS('',3,(#37434,#37435,#37436,#37437,#37438,
#37439,#37440,#37441,#37442,#37443),.UNSPECIFIED.,.F.,.F.,(4,2,2,2,4),(0.,
0.225488637846501,0.450977275693002,0.705434126471363,0.959890977249723),
 .UNSPECIFIED.);
#10982=B_SPLINE_CURVE_WITH_KNOTS('',3,(#37447,#37448,#37449,#37450,#37451,
#37452,#37453,#37454,#37455,#37456),.UNSPECIFIED.,.F.,.F.,(4,2,2,2,4),(0.944884480326527,
1.19934133110489,1.45379818188325,1.67928681972975,1.90477545757625),
 .UNSPECIFIED.);
#10983=B_SPLINE_CURVE_WITH_KNOTS('',3,(#37460,#37461,#37462,#37463,#37464,
#37465,#37466,#37467,#37468,#37469),.UNSPECIFIED.,.F.,.F.,(4,2,2,2,4),(1.9047986617354,
2.1302872995819,2.35577593742841,2.61023278820676,2.86468963898512),
 .UNSPECIFIED.);
#10984=B_SPLINE_CURVE_WITH_KNOTS('',3,(#37473,#37474,#37475,#37476,#37477,
#37478,#37479,#37480,#37481,#37482),.UNSPECIFIED.,.F.,.F.,(4,2,2,2,4),(-0.33267099144991,
-0.240960064975725,-0.149249138501539,-0.0746245692507697,0.),
 .UNSPECIFIED.);
#10985=B_SPLINE_CURVE_WITH_KNOTS('',3,(#37485,#37486,#37487,#37488,#37489,
#37490),.UNSPECIFIED.,.F.,.F.,(4,2,4),(0.668371667822993,0.742996237073762,
0.770694061397097),.UNSPECIFIED.);
#10986=B_SPLINE_CURVE_WITH_KNOTS('',3,(#37942,#37943,#37944,#37945,#37946,
#37947,#37948,#37949,#37950,#37951),.UNSPECIFIED.,.F.,.F.,(4,2,2,2,4),(0.,
0.0753377480935412,0.150675496187082,0.226025649710019,0.301375803232956),
 .UNSPECIFIED.);
#10987=B_SPLINE_CURVE_WITH_KNOTS('',3,(#37955,#37956,#37957,#37958,#37959,
#37960,#37961,#37962,#37963,#37964),.UNSPECIFIED.,.F.,.F.,(4,2,2,2,4),(-0.301375803232957,
-0.226025649710019,-0.150675496187082,-0.0753377480935411,0.),
 .UNSPECIFIED.);
#10988=B_SPLINE_CURVE_WITH_KNOTS('',3,(#37987,#37988,#37989,#37990,#37991,
#37992,#37993,#37994,#37995,#37996,#37997,#37998,#37999,#38000),
 .UNSPECIFIED.,.F.,.F.,(4,2,2,2,2,2,4),(-0.00091047155368565,0.,0.0913567345993141,
0.177776562764162,0.263923329391251,0.328582398254389,0.38525018680505),
 .UNSPECIFIED.);
#10989=B_SPLINE_CURVE_WITH_KNOTS('',3,(#38004,#38005,#38006,#38007,#38008,
#38009,#38010,#38011,#38012,#38013,#38014,#38015,#38016,#38017),
 .UNSPECIFIED.,.F.,.F.,(4,2,2,2,2,2,4),(-0.771410845200401,-0.770500373646599,
-0.679143639043445,-0.592723810874369,-0.506577044243045,-0.441917975376721,
-0.38525018682332),.UNSPECIFIED.);
#10990=B_SPLINE_CURVE_WITH_KNOTS('',3,(#38092,#38093,#38094,#38095,#38096,
#38097,#38098,#38099),.UNSPECIFIED.,.F.,.F.,(4,1,1,1,1,4),(-1.86233569221144,
-1.59628773618123,-1.06419182412082,-0.798143868090616,-0.532095912060411,
0.),.UNSPECIFIED.);
#10991=B_SPLINE_CURVE_WITH_KNOTS('',3,(#38100,#38101,#38102,#38103,#38104,
#38105,#38106,#38107),.UNSPECIFIED.,.F.,.F.,(4,1,1,1,1,4),(0.,0.532095912060411,
0.798143868090616,1.06419182412082,1.59628773618123,1.86233569221144),
 .UNSPECIFIED.);
#10992=B_SPLINE_CURVE_WITH_KNOTS('',3,(#38162,#38163,#38164,#38165,#38166,
#38167,#38168,#38169),.UNSPECIFIED.,.F.,.F.,(4,1,1,1,1,4),(-1.8623356922078,
-1.33023978014843,-1.06419182411875,-0.798143868089059,-0.532095912059373,
-8.87358627225765E-17),.UNSPECIFIED.);
#10993=B_SPLINE_CURVE_WITH_KNOTS('',3,(#38170,#38171,#38172,#38173,#38174,
#38175,#38176,#38177),.UNSPECIFIED.,.F.,.F.,(4,1,1,1,1,4),(8.87358627225765E-17,
0.532095912059373,0.798143868089059,1.06419182411875,1.33023978014843,1.8623356922078),
 .UNSPECIFIED.);
#10994=B_SPLINE_CURVE_WITH_KNOTS('',3,(#38231,#38232,#38233,#38234,#38235,
#38236,#38237,#38238,#38239),.UNSPECIFIED.,.F.,.F.,(4,1,1,1,1,1,4),(-1.86233569221144,
-1.46326375816613,-1.33023978015103,-1.06419182412082,-0.798143868090615,
-0.266047956030205,0.),.UNSPECIFIED.);
#10995=B_SPLINE_CURVE_WITH_KNOTS('',3,(#38369,#38370,#38371,#38372,#38373,
#38374,#38375,#38376,#38377),.UNSPECIFIED.,.F.,.F.,(4,1,1,1,1,1,4),(0.,
0.266047956030205,0.798143868090615,1.06419182412082,1.33023978015103,1.46326375816613,
1.86233569221144),.UNSPECIFIED.);
#10996=B_SPLINE_CURVE_WITH_KNOTS('',3,(#38432,#38433,#38434,#38435,#38436,
#38437,#38438,#38439),.UNSPECIFIED.,.F.,.F.,(4,1,1,1,1,4),(-1.86233569220781,
-1.59628773617812,-1.06419182411875,-0.79814386808906,-0.532095912059373,
-2.59005157847017E-16),.UNSPECIFIED.);
#10997=B_SPLINE_CURVE_WITH_KNOTS('',3,(#38440,#38441,#38442,#38443,#38444,
#38445,#38446,#38447),.UNSPECIFIED.,.F.,.F.,(4,1,1,1,1,4),(2.59005157847017E-16,
0.532095912059373,0.79814386808906,1.06419182411875,1.59628773617812,1.86233569220781),
 .UNSPECIFIED.);
#11462=VERTEX_POINT('',#37378);
#11463=VERTEX_POINT('',#37379);
#11464=VERTEX_POINT('',#37386);
#11465=VERTEX_POINT('',#37388);
#11466=VERTEX_POINT('',#37391);
#11467=VERTEX_POINT('',#37393);
#11468=VERTEX_POINT('',#37414);
#11469=VERTEX_POINT('',#37416);
#11470=VERTEX_POINT('',#37418);
#11471=VERTEX_POINT('',#37420);
#11472=VERTEX_POINT('',#37431);
#11473=VERTEX_POINT('',#37433);
#11474=VERTEX_POINT('',#37444);
#11475=VERTEX_POINT('',#37446);
#11476=VERTEX_POINT('',#37457);
#11477=VERTEX_POINT('',#37459);
#11478=VERTEX_POINT('',#37470);
#11479=VERTEX_POINT('',#37472);
#11480=VERTEX_POINT('',#37483);
#11481=VERTEX_POINT('',#37492);
#11482=VERTEX_POINT('',#37494);
#11483=VERTEX_POINT('',#37496);
#11484=VERTEX_POINT('',#37498);
#11485=VERTEX_POINT('',#37500);
#11486=VERTEX_POINT('',#37503);
#11487=VERTEX_POINT('',#37509);
#11488=VERTEX_POINT('',#37511);
#11489=VERTEX_POINT('',#37513);
#11490=VERTEX_POINT('',#37515);
#11491=VERTEX_POINT('',#37517);
#11492=VERTEX_POINT('',#37519);
#11493=VERTEX_POINT('',#37521);
#11494=VERTEX_POINT('',#37523);
#11495=VERTEX_POINT('',#37525);
#11496=VERTEX_POINT('',#37528);
#11497=VERTEX_POINT('',#37529);
#11498=VERTEX_POINT('',#37531);
#11499=VERTEX_POINT('',#37533);
#11500=VERTEX_POINT('',#37545);
#11501=VERTEX_POINT('',#37546);
#11502=VERTEX_POINT('',#37551);
#11503=VERTEX_POINT('',#37552);
#11504=VERTEX_POINT('',#37565);
#11505=VERTEX_POINT('',#37566);
#11506=VERTEX_POINT('',#37571);
#11507=VERTEX_POINT('',#37572);
#11508=VERTEX_POINT('',#37585);
#11509=VERTEX_POINT('',#37586);
#11510=VERTEX_POINT('',#37591);
#11511=VERTEX_POINT('',#37592);
#11512=VERTEX_POINT('',#37608);
#11513=VERTEX_POINT('',#37610);
#11514=VERTEX_POINT('',#37614);
#11515=VERTEX_POINT('',#37618);
#11516=VERTEX_POINT('',#37622);
#11517=VERTEX_POINT('',#37626);
#11518=VERTEX_POINT('',#37628);
#11519=VERTEX_POINT('',#37631);
#11520=VERTEX_POINT('',#37632);
#11521=VERTEX_POINT('',#37634);
#11522=VERTEX_POINT('',#37636);
#11523=VERTEX_POINT('',#37648);
#11524=VERTEX_POINT('',#37649);
#11525=VERTEX_POINT('',#37654);
#11526=VERTEX_POINT('',#37667);
#11527=VERTEX_POINT('',#37671);
#11528=VERTEX_POINT('',#37683);
#11529=VERTEX_POINT('',#37687);
#11530=VERTEX_POINT('',#37708);
#11531=VERTEX_POINT('',#37709);
#11532=VERTEX_POINT('',#37711);
#11533=VERTEX_POINT('',#37713);
#11534=VERTEX_POINT('',#37715);
#11535=VERTEX_POINT('',#37717);
#11536=VERTEX_POINT('',#37719);
#11537=VERTEX_POINT('',#37721);
#11538=VERTEX_POINT('',#37724);
#11539=VERTEX_POINT('',#37726);
#11540=VERTEX_POINT('',#37729);
#11541=VERTEX_POINT('',#37730);
#11542=VERTEX_POINT('',#37732);
#11543=VERTEX_POINT('',#37734);
#11544=VERTEX_POINT('',#37746);
#11545=VERTEX_POINT('',#37747);
#11546=VERTEX_POINT('',#37752);
#11547=VERTEX_POINT('',#37753);
#11548=VERTEX_POINT('',#37766);
#11549=VERTEX_POINT('',#37767);
#11550=VERTEX_POINT('',#37772);
#11551=VERTEX_POINT('',#37773);
#11552=VERTEX_POINT('',#37786);
#11553=VERTEX_POINT('',#37787);
#11554=VERTEX_POINT('',#37792);
#11555=VERTEX_POINT('',#37793);
#11556=VERTEX_POINT('',#37809);
#11557=VERTEX_POINT('',#37811);
#11558=VERTEX_POINT('',#37815);
#11559=VERTEX_POINT('',#37819);
#11560=VERTEX_POINT('',#37823);
#11561=VERTEX_POINT('',#37827);
#11562=VERTEX_POINT('',#37830);
#11563=VERTEX_POINT('',#37831);
#11564=VERTEX_POINT('',#37833);
#11565=VERTEX_POINT('',#37835);
#11566=VERTEX_POINT('',#37847);
#11567=VERTEX_POINT('',#37848);
#11568=VERTEX_POINT('',#37853);
#11569=VERTEX_POINT('',#37854);
#11570=VERTEX_POINT('',#37867);
#11571=VERTEX_POINT('',#37868);
#11572=VERTEX_POINT('',#37873);
#11573=VERTEX_POINT('',#37874);
#11574=VERTEX_POINT('',#37887);
#11575=VERTEX_POINT('',#37888);
#11576=VERTEX_POINT('',#37893);
#11577=VERTEX_POINT('',#37894);
#11578=VERTEX_POINT('',#37910);
#11579=VERTEX_POINT('',#37912);
#11580=VERTEX_POINT('',#37916);
#11581=VERTEX_POINT('',#37920);
#11582=VERTEX_POINT('',#37924);
#11583=VERTEX_POINT('',#37928);
#11584=VERTEX_POINT('',#37931);
#11585=VERTEX_POINT('',#37935);
#11586=VERTEX_POINT('',#37937);
#11587=VERTEX_POINT('',#37939);
#11588=VERTEX_POINT('',#37941);
#11589=VERTEX_POINT('',#37952);
#11590=VERTEX_POINT('',#37954);
#11591=VERTEX_POINT('',#37965);
#11592=VERTEX_POINT('',#37969);
#11593=VERTEX_POINT('',#37971);
#11594=VERTEX_POINT('',#37975);
#11595=VERTEX_POINT('',#37977);
#11596=VERTEX_POINT('',#37981);
#11597=VERTEX_POINT('',#37985);
#11598=VERTEX_POINT('',#38002);
#11599=VERTEX_POINT('',#38021);
#11600=VERTEX_POINT('',#38025);
#11601=VERTEX_POINT('',#38031);
#11602=VERTEX_POINT('',#38032);
#11603=VERTEX_POINT('',#38034);
#11604=VERTEX_POINT('',#38036);
#11605=VERTEX_POINT('',#38038);
#11606=VERTEX_POINT('',#38089);
#11607=VERTEX_POINT('',#38090);
#11608=VERTEX_POINT('',#38109);
#11609=VERTEX_POINT('',#38110);
#11610=VERTEX_POINT('',#38179);
#11611=VERTEX_POINT('',#38181);
#11612=VERTEX_POINT('',#38183);
#11613=VERTEX_POINT('',#38185);
#11614=VERTEX_POINT('',#38189);
#11615=VERTEX_POINT('',#38193);
#11616=VERTEX_POINT('',#38197);
#11617=VERTEX_POINT('',#38199);
#11618=VERTEX_POINT('',#38203);
#11619=VERTEX_POINT('',#38204);
#11620=VERTEX_POINT('',#38206);
#11621=VERTEX_POINT('',#38208);
#11622=VERTEX_POINT('',#38212);
#11623=VERTEX_POINT('',#38213);
#11624=VERTEX_POINT('',#38224);
#11625=VERTEX_POINT('',#38226);
#11626=VERTEX_POINT('',#38228);
#11627=VERTEX_POINT('',#38230);
#11628=VERTEX_POINT('',#38246);
#11629=VERTEX_POINT('',#38247);
#11630=VERTEX_POINT('',#38250);
#11631=VERTEX_POINT('',#38254);
#11632=VERTEX_POINT('',#38258);
#11633=VERTEX_POINT('',#38262);
#11634=VERTEX_POINT('',#38266);
#11635=VERTEX_POINT('',#38270);
#11636=VERTEX_POINT('',#38271);
#11637=VERTEX_POINT('',#38276);
#11638=VERTEX_POINT('',#38277);
#11639=VERTEX_POINT('',#38285);
#11640=VERTEX_POINT('',#38289);
#11641=VERTEX_POINT('',#38291);
#11642=VERTEX_POINT('',#38293);
#11643=VERTEX_POINT('',#38296);
#11644=VERTEX_POINT('',#38298);
#11645=VERTEX_POINT('',#38300);
#11646=VERTEX_POINT('',#38303);
#11647=VERTEX_POINT('',#38306);
#11648=VERTEX_POINT('',#38308);
#11649=VERTEX_POINT('',#38310);
#11650=VERTEX_POINT('',#38367);
#11651=VERTEX_POINT('',#38379);
#11652=VERTEX_POINT('',#38380);
#11653=VERTEX_POINT('',#38452);
#11654=VERTEX_POINT('',#38460);
#11655=VERTEX_POINT('',#38465);
#11656=VERTEX_POINT('',#38470);
#11657=VERTEX_POINT('',#38478);
#11658=VERTEX_POINT('',#38482);
#11659=VERTEX_POINT('',#38487);
#11660=VERTEX_POINT('',#38492);
#11661=VERTEX_POINT('',#38497);
#11662=VERTEX_POINT('',#38502);
#11663=VERTEX_POINT('',#38507);
#11664=VERTEX_POINT('',#38512);
#11665=VERTEX_POINT('',#38517);
#11666=VERTEX_POINT('',#38522);
#11667=VERTEX_POINT('',#38527);
#11668=VERTEX_POINT('',#38532);
#11669=VERTEX_POINT('',#38537);
#11670=VERTEX_POINT('',#38543);
#11671=VERTEX_POINT('',#38579);
#13905=EDGE_CURVE('',#11462,#11463,#10978,.F.);
#13906=EDGE_CURVE('',#11463,#11464,#10119,.T.);
#13907=EDGE_CURVE('',#11464,#11465,#10120,.T.);
#13908=EDGE_CURVE('',#11465,#11465,#10121,.T.);
#13909=EDGE_CURVE('',#11464,#11466,#10122,.T.);
#13910=EDGE_CURVE('',#11466,#11467,#10979,.F.);
#13911=EDGE_CURVE('',#11462,#11467,#10123,.T.);
#13912=EDGE_CURVE('',#11463,#11468,#1758,.T.);
#13913=EDGE_CURVE('',#11469,#11468,#10124,.T.);
#13914=EDGE_CURVE('',#11470,#11469,#10125,.T.);
#13915=EDGE_CURVE('',#11470,#11471,#10980,.T.);
#13916=EDGE_CURVE('',#11471,#11472,#1759,.T.);
#13917=EDGE_CURVE('',#11472,#11473,#10981,.T.);
#13918=EDGE_CURVE('',#11473,#11474,#10126,.T.);
#13919=EDGE_CURVE('',#11474,#11475,#10982,.T.);
#13920=EDGE_CURVE('',#11475,#11476,#1760,.T.);
#13921=EDGE_CURVE('',#11476,#11477,#10983,.T.);
#13922=EDGE_CURVE('',#11478,#11477,#10127,.T.);
#13923=EDGE_CURVE('',#11479,#11478,#10984,.F.);
#13924=EDGE_CURVE('',#11479,#11480,#1761,.T.);
#13925=EDGE_CURVE('',#11466,#11480,#10985,.F.);
#13926=EDGE_CURVE('',#11481,#11481,#10128,.T.);
#13927=EDGE_CURVE('',#11482,#11482,#10129,.T.);
#13928=EDGE_CURVE('',#11483,#11483,#10130,.T.);
#13929=EDGE_CURVE('',#11484,#11484,#10131,.T.);
#13930=EDGE_CURVE('',#11485,#11485,#10132,.T.);
#13931=EDGE_CURVE('',#11469,#11486,#10133,.T.);
#13932=EDGE_CURVE('',#11486,#11486,#10134,.T.);
#13933=EDGE_CURVE('',#11468,#11478,#10135,.T.);
#13934=EDGE_CURVE('',#11477,#11470,#10136,.T.);
#13935=EDGE_CURVE('',#11487,#11487,#10137,.T.);
#13936=EDGE_CURVE('',#11488,#11488,#10138,.T.);
#13937=EDGE_CURVE('',#11489,#11489,#10139,.T.);
#13938=EDGE_CURVE('',#11490,#11490,#10140,.T.);
#13939=EDGE_CURVE('',#11491,#11491,#10141,.T.);
#13940=EDGE_CURVE('',#11492,#11492,#10142,.T.);
#13941=EDGE_CURVE('',#11493,#11493,#10143,.T.);
#13942=EDGE_CURVE('',#11494,#11494,#10144,.T.);
#13943=EDGE_CURVE('',#11495,#11495,#10145,.T.);
#13944=EDGE_CURVE('',#11496,#11497,#10146,.T.);
#13945=EDGE_CURVE('',#11497,#11498,#1762,.T.);
#13946=EDGE_CURVE('',#11498,#11499,#10147,.T.);
#13947=EDGE_CURVE('',#11499,#11496,#1763,.T.);
#13948=EDGE_CURVE('',#11500,#11501,#10148,.T.);
#13949=EDGE_CURVE('',#11501,#11499,#10149,.T.);
#13950=EDGE_CURVE('',#11498,#11500,#10150,.T.);
#13951=EDGE_CURVE('',#11502,#11503,#10151,.T.);
#13952=EDGE_CURVE('',#11503,#11501,#1764,.T.);
#13953=EDGE_CURVE('',#11500,#11502,#1765,.T.);
#13954=EDGE_CURVE('',#11504,#11505,#10152,.T.);
#13955=EDGE_CURVE('',#11505,#11503,#10153,.T.);
#13956=EDGE_CURVE('',#11502,#11504,#10154,.T.);
#13957=EDGE_CURVE('',#11506,#11507,#10155,.T.);
#13958=EDGE_CURVE('',#11507,#11505,#1766,.T.);
#13959=EDGE_CURVE('',#11504,#11506,#1767,.T.);
#13960=EDGE_CURVE('',#11508,#11509,#10156,.T.);
#13961=EDGE_CURVE('',#11509,#11507,#10157,.T.);
#13962=EDGE_CURVE('',#11506,#11508,#10158,.T.);
#13963=EDGE_CURVE('',#11510,#11511,#10159,.T.);
#13964=EDGE_CURVE('',#11511,#11509,#1768,.T.);
#13965=EDGE_CURVE('',#11508,#11510,#1769,.T.);
#13966=EDGE_CURVE('',#11496,#11511,#10160,.T.);
#13967=EDGE_CURVE('',#11510,#11497,#10161,.T.);
#13968=EDGE_CURVE('',#11509,#11512,#1770,.T.);
#13969=EDGE_CURVE('',#11513,#11512,#10162,.T.);
#13970=EDGE_CURVE('',#11507,#11513,#1771,.T.);
#13971=EDGE_CURVE('',#11511,#11514,#1772,.T.);
#13972=EDGE_CURVE('',#11512,#11514,#1773,.T.);
#13973=EDGE_CURVE('',#11496,#11515,#1774,.T.);
#13974=EDGE_CURVE('',#11514,#11515,#10163,.T.);
#13975=EDGE_CURVE('',#11499,#11516,#1775,.T.);
#13976=EDGE_CURVE('',#11515,#11516,#1776,.T.);
#13977=EDGE_CURVE('',#11517,#11517,#10164,.T.);
#13978=EDGE_CURVE('',#11518,#11518,#10165,.T.);
#13979=EDGE_CURVE('',#11519,#11520,#10166,.T.);
#13980=EDGE_CURVE('',#11520,#11521,#1777,.T.);
#13981=EDGE_CURVE('',#11521,#11522,#10167,.T.);
#13982=EDGE_CURVE('',#11522,#11519,#1778,.T.);
#13983=EDGE_CURVE('',#11523,#11524,#10168,.T.);
#13984=EDGE_CURVE('',#11524,#11522,#10169,.T.);
#13985=EDGE_CURVE('',#11521,#11523,#10170,.T.);
#13986=EDGE_CURVE('',#11513,#11525,#10171,.T.);
#13987=EDGE_CURVE('',#11525,#11524,#1779,.T.);
#13988=EDGE_CURVE('',#11523,#11513,#1780,.T.);
#13989=EDGE_CURVE('',#11512,#11526,#10172,.T.);
#13990=EDGE_CURVE('',#11526,#11525,#10173,.T.);
#13991=EDGE_CURVE('',#11514,#11527,#10174,.T.);
#13992=EDGE_CURVE('',#11527,#11526,#1781,.T.);
#13993=EDGE_CURVE('',#11515,#11528,#10175,.T.);
#13994=EDGE_CURVE('',#11528,#11527,#10176,.T.);
#13995=EDGE_CURVE('',#11516,#11529,#10177,.T.);
#13996=EDGE_CURVE('',#11529,#11528,#1782,.T.);
#13997=EDGE_CURVE('',#11519,#11529,#10178,.T.);
#13998=EDGE_CURVE('',#11516,#11520,#10179,.T.);
#13999=EDGE_CURVE('',#11505,#11523,#1783,.T.);
#14000=EDGE_CURVE('',#11503,#11521,#1784,.T.);
#14001=EDGE_CURVE('',#11501,#11520,#1785,.T.);
#14002=EDGE_CURVE('',#11530,#11531,#10180,.T.);
#14003=EDGE_CURVE('',#11532,#11530,#1786,.T.);
#14004=EDGE_CURVE('',#11533,#11532,#10181,.T.);
#14005=EDGE_CURVE('',#11534,#11533,#1787,.T.);
#14006=EDGE_CURVE('',#11535,#11534,#10182,.T.);
#14007=EDGE_CURVE('',#11536,#11535,#1788,.T.);
#14008=EDGE_CURVE('',#11537,#11536,#10183,.T.);
#14009=EDGE_CURVE('',#11531,#11537,#1789,.T.);
#14010=EDGE_CURVE('',#11538,#11538,#10184,.T.);
#14011=EDGE_CURVE('',#11539,#11539,#10185,.T.);
#14012=EDGE_CURVE('',#11540,#11541,#10186,.T.);
#14013=EDGE_CURVE('',#11541,#11542,#1790,.T.);
#14014=EDGE_CURVE('',#11542,#11543,#10187,.T.);
#14015=EDGE_CURVE('',#11543,#11540,#1791,.T.);
#14016=EDGE_CURVE('',#11544,#11545,#10188,.T.);
#14017=EDGE_CURVE('',#11545,#11543,#10189,.T.);
#14018=EDGE_CURVE('',#11542,#11544,#10190,.T.);
#14019=EDGE_CURVE('',#11546,#11547,#10191,.T.);
#14020=EDGE_CURVE('',#11547,#11545,#1792,.T.);
#14021=EDGE_CURVE('',#11544,#11546,#1793,.T.);
#14022=EDGE_CURVE('',#11548,#11549,#10192,.T.);
#14023=EDGE_CURVE('',#11549,#11547,#10193,.T.);
#14024=EDGE_CURVE('',#11546,#11548,#10194,.T.);
#14025=EDGE_CURVE('',#11550,#11551,#10195,.T.);
#14026=EDGE_CURVE('',#11551,#11549,#1794,.T.);
#14027=EDGE_CURVE('',#11548,#11550,#1795,.T.);
#14028=EDGE_CURVE('',#11552,#11553,#10196,.T.);
#14029=EDGE_CURVE('',#11553,#11551,#10197,.T.);
#14030=EDGE_CURVE('',#11550,#11552,#10198,.T.);
#14031=EDGE_CURVE('',#11554,#11555,#10199,.T.);
#14032=EDGE_CURVE('',#11555,#11553,#1796,.T.);
#14033=EDGE_CURVE('',#11552,#11554,#1797,.T.);
#14034=EDGE_CURVE('',#11540,#11555,#10200,.T.);
#14035=EDGE_CURVE('',#11554,#11541,#10201,.T.);
#14036=EDGE_CURVE('',#11556,#11546,#1798,.T.);
#14037=EDGE_CURVE('',#11557,#11556,#10202,.T.);
#14038=EDGE_CURVE('',#11557,#11548,#1799,.T.);
#14039=EDGE_CURVE('',#11558,#11544,#1800,.T.);
#14040=EDGE_CURVE('',#11556,#11558,#1801,.T.);
#14041=EDGE_CURVE('',#11559,#11542,#1802,.T.);
#14042=EDGE_CURVE('',#11558,#11559,#10203,.T.);
#14043=EDGE_CURVE('',#11560,#11541,#1803,.T.);
#14044=EDGE_CURVE('',#11559,#11560,#1804,.T.);
#14045=EDGE_CURVE('',#11561,#11561,#10204,.T.);
#14046=EDGE_CURVE('',#11562,#11563,#10205,.T.);
#14047=EDGE_CURVE('',#11563,#11564,#1805,.T.);
#14048=EDGE_CURVE('',#11564,#11565,#10206,.T.);
#14049=EDGE_CURVE('',#11565,#11562,#1806,.T.);
#14050=EDGE_CURVE('',#11566,#11567,#10207,.T.);
#14051=EDGE_CURVE('',#11567,#11565,#10208,.T.);
#14052=EDGE_CURVE('',#11564,#11566,#10209,.T.);
#14053=EDGE_CURVE('',#11568,#11569,#10210,.T.);
#14054=EDGE_CURVE('',#11569,#11567,#1807,.T.);
#14055=EDGE_CURVE('',#11566,#11568,#1808,.T.);
#14056=EDGE_CURVE('',#11570,#11571,#10211,.T.);
#14057=EDGE_CURVE('',#11571,#11569,#10212,.T.);
#14058=EDGE_CURVE('',#11568,#11570,#10213,.T.);
#14059=EDGE_CURVE('',#11572,#11573,#10214,.T.);
#14060=EDGE_CURVE('',#11573,#11571,#1809,.T.);
#14061=EDGE_CURVE('',#11570,#11572,#1810,.T.);
#14062=EDGE_CURVE('',#11574,#11575,#10215,.T.);
#14063=EDGE_CURVE('',#11575,#11573,#10216,.T.);
#14064=EDGE_CURVE('',#11572,#11574,#10217,.T.);
#14065=EDGE_CURVE('',#11576,#11577,#10218,.T.);
#14066=EDGE_CURVE('',#11577,#11575,#1811,.T.);
#14067=EDGE_CURVE('',#11574,#11576,#1812,.T.);
#14068=EDGE_CURVE('',#11562,#11577,#10219,.T.);
#14069=EDGE_CURVE('',#11576,#11563,#10220,.T.);
#14070=EDGE_CURVE('',#11578,#11568,#1813,.T.);
#14071=EDGE_CURVE('',#11579,#11578,#10221,.T.);
#14072=EDGE_CURVE('',#11579,#11570,#1814,.T.);
#14073=EDGE_CURVE('',#11580,#11566,#1815,.T.);
#14074=EDGE_CURVE('',#11578,#11580,#1816,.T.);
#14075=EDGE_CURVE('',#11581,#11564,#1817,.T.);
#14076=EDGE_CURVE('',#11580,#11581,#10222,.T.);
#14077=EDGE_CURVE('',#11582,#11563,#1818,.T.);
#14078=EDGE_CURVE('',#11581,#11582,#1819,.T.);
#14079=EDGE_CURVE('',#11583,#11583,#10223,.T.);
#14080=EDGE_CURVE('',#11495,#11584,#10224,.T.);
#14081=EDGE_CURVE('',#11584,#11584,#10225,.T.);
#14082=EDGE_CURVE('',#11584,#11585,#1820,.T.);
#14083=EDGE_CURVE('',#11585,#11586,#10226,.T.);
#14084=EDGE_CURVE('',#11587,#11586,#1821,.T.);
#14085=EDGE_CURVE('',#11588,#11587,#10986,.F.);
#14086=EDGE_CURVE('',#11588,#11589,#10227,.T.);
#14087=EDGE_CURVE('',#11590,#11589,#10987,.F.);
#14088=EDGE_CURVE('',#11590,#11591,#1822,.T.);
#14089=EDGE_CURVE('',#11591,#11585,#10228,.T.);
#14090=EDGE_CURVE('',#11592,#11592,#10229,.T.);
#14091=EDGE_CURVE('',#11592,#11593,#10230,.T.);
#14092=EDGE_CURVE('',#11593,#11593,#10231,.T.);
#14093=EDGE_CURVE('',#11589,#11594,#1823,.T.);
#14094=EDGE_CURVE('',#11595,#11588,#1824,.T.);
#14095=EDGE_CURVE('',#11594,#11595,#10232,.T.);
#14096=EDGE_CURVE('',#11593,#11596,#1825,.T.);
#14097=EDGE_CURVE('',#11596,#11596,#10233,.T.);
#14098=EDGE_CURVE('',#11597,#11590,#1826,.T.);
#14099=EDGE_CURVE('',#11594,#11597,#10988,.T.);
#14100=EDGE_CURVE('',#11598,#11597,#10234,.T.);
#14101=EDGE_CURVE('',#11595,#11598,#10989,.T.);
#14102=EDGE_CURVE('',#11587,#11598,#1827,.T.);
#14103=EDGE_CURVE('',#11597,#11599,#1828,.T.);
#14104=EDGE_CURVE('',#11599,#11591,#1829,.T.);
#14105=EDGE_CURVE('',#11598,#11600,#1830,.T.);
#14106=EDGE_CURVE('',#11600,#11599,#10235,.T.);
#14107=EDGE_CURVE('',#11586,#11600,#1831,.T.);
#14108=EDGE_CURVE('',#11601,#11602,#10236,.T.);
#14109=EDGE_CURVE('',#11602,#11603,#10237,.T.);
#14110=EDGE_CURVE('',#11603,#11604,#10238,.T.);
#14111=EDGE_CURVE('',#11604,#11605,#10239,.T.);
#14112=EDGE_CURVE('',#11605,#11601,#10240,.T.);
#14113=EDGE_CURVE('',#11606,#11607,#10241,.T.);
#14114=EDGE_CURVE('',#11607,#11605,#10990,.T.);
#14115=EDGE_CURVE('',#11604,#11606,#10991,.T.);
#14116=EDGE_CURVE('',#11608,#11609,#10242,.T.);
#14117=EDGE_CURVE('',#11609,#11607,#10243,.T.);
#14118=EDGE_CURVE('',#11606,#11608,#10244,.T.);
#14119=EDGE_CURVE('',#11601,#11609,#10992,.T.);
#14120=EDGE_CURVE('',#11608,#11602,#10993,.T.);
#14121=EDGE_CURVE('',#11601,#11610,#1832,.T.);
#14122=EDGE_CURVE('',#11611,#11610,#10245,.T.);
#14123=EDGE_CURVE('',#11612,#11611,#1833,.T.);
#14124=EDGE_CURVE('',#11612,#11613,#10246,.T.);
#14125=EDGE_CURVE('',#11613,#11609,#1834,.T.);
#14126=EDGE_CURVE('',#11605,#11614,#1835,.T.);
#14127=EDGE_CURVE('',#11610,#11614,#1836,.T.);
#14128=EDGE_CURVE('',#11603,#11615,#1837,.T.);
#14129=EDGE_CURVE('',#11615,#11615,#10247,.T.);
#14130=EDGE_CURVE('',#11480,#11616,#1838,.T.);
#14131=EDGE_CURVE('',#11616,#11617,#10248,.T.);
#14132=EDGE_CURVE('',#11617,#11467,#1839,.T.);
#14133=EDGE_CURVE('',#11618,#11619,#10249,.T.);
#14134=EDGE_CURVE('',#11619,#11620,#1840,.T.);
#14135=EDGE_CURVE('',#11620,#11621,#10250,.T.);
#14136=EDGE_CURVE('',#11621,#11618,#1841,.T.);
#14137=EDGE_CURVE('',#11622,#11623,#10251,.T.);
#14138=EDGE_CURVE('',#11623,#11621,#10252,.T.);
#14139=EDGE_CURVE('',#11620,#11622,#10253,.T.);
#14140=EDGE_CURVE('',#11478,#11623,#1842,.T.);
#14141=EDGE_CURVE('',#11622,#11479,#1843,.T.);
#14142=EDGE_CURVE('',#11618,#11617,#10254,.T.);
#14143=EDGE_CURVE('',#11616,#11619,#10255,.T.);
#14144=EDGE_CURVE('',#11623,#11624,#1844,.T.);
#14145=EDGE_CURVE('',#11625,#11624,#10256,.T.);
#14146=EDGE_CURVE('',#11626,#11625,#1845,.T.);
#14147=EDGE_CURVE('',#11627,#11626,#10994,.T.);
#14148=EDGE_CURVE('',#11621,#11627,#1846,.T.);
#14149=EDGE_CURVE('',#11468,#11612,#1847,.T.);
#14150=EDGE_CURVE('',#11624,#11611,#1848,.T.);
#14151=EDGE_CURVE('',#11628,#11629,#10257,.T.);
#14152=EDGE_CURVE('',#11629,#11625,#1849,.T.);
#14153=EDGE_CURVE('',#11625,#11630,#10258,.T.);
#14154=EDGE_CURVE('',#11630,#11628,#1850,.T.);
#14155=EDGE_CURVE('',#11624,#11631,#10259,.T.);
#14156=EDGE_CURVE('',#11631,#11630,#10260,.T.);
#14157=EDGE_CURVE('',#11611,#11632,#10261,.T.);
#14158=EDGE_CURVE('',#11632,#11631,#1851,.T.);
#14159=EDGE_CURVE('',#11610,#11633,#10262,.T.);
#14160=EDGE_CURVE('',#11633,#11632,#10263,.T.);
#14161=EDGE_CURVE('',#11614,#11634,#10264,.T.);
#14162=EDGE_CURVE('',#11634,#11633,#1852,.T.);
#14163=EDGE_CURVE('',#11635,#11636,#10265,.T.);
#14164=EDGE_CURVE('',#11636,#11634,#10266,.T.);
#14165=EDGE_CURVE('',#11614,#11635,#10267,.T.);
#14166=EDGE_CURVE('',#11637,#11638,#10268,.T.);
#14167=EDGE_CURVE('',#11638,#11636,#1853,.T.);
#14168=EDGE_CURVE('',#11635,#11637,#1854,.T.);
#14169=EDGE_CURVE('',#11628,#11638,#10269,.T.);
#14170=EDGE_CURVE('',#11637,#11629,#10270,.T.);
#14171=EDGE_CURVE('',#11639,#11629,#1855,.T.);
#14172=EDGE_CURVE('',#11626,#11639,#10271,.T.);
#14173=EDGE_CURVE('',#11560,#11640,#10272,.T.);
#14174=EDGE_CURVE('',#11640,#11641,#1856,.T.);
#14175=EDGE_CURVE('',#11641,#11642,#10273,.T.);
#14176=EDGE_CURVE('',#11642,#11557,#1857,.T.);
#14177=EDGE_CURVE('',#11582,#11643,#10274,.T.);
#14178=EDGE_CURVE('',#11643,#11644,#1858,.T.);
#14179=EDGE_CURVE('',#11644,#11645,#10275,.T.);
#14180=EDGE_CURVE('',#11645,#11579,#1859,.T.);
#14181=EDGE_CURVE('',#11646,#11646,#10276,.T.);
#14182=EDGE_CURVE('',#11639,#11647,#10277,.T.);
#14183=EDGE_CURVE('',#11647,#11648,#10278,.T.);
#14184=EDGE_CURVE('',#11648,#11649,#10279,.T.);
#14185=EDGE_CURVE('',#11649,#11626,#10280,.T.);
#14186=EDGE_CURVE('',#11650,#11627,#10281,.T.);
#14187=EDGE_CURVE('',#11649,#11650,#10995,.T.);
#14188=EDGE_CURVE('',#11651,#11652,#10282,.T.);
#14189=EDGE_CURVE('',#11652,#11627,#10283,.T.);
#14190=EDGE_CURVE('',#11650,#11651,#10284,.T.);
#14191=EDGE_CURVE('',#11639,#11652,#10996,.T.);
#14192=EDGE_CURVE('',#11651,#11647,#10997,.T.);
#14193=EDGE_CURVE('',#11618,#11652,#1860,.T.);
#14194=EDGE_CURVE('',#11617,#11637,#1861,.T.);
#14195=EDGE_CURVE('',#11648,#11653,#1862,.T.);
#14196=EDGE_CURVE('',#11653,#11653,#10285,.T.);
#14197=EDGE_CURVE('',#11539,#11518,#1863,.T.);
#14198=EDGE_CURVE('',#11538,#11517,#1864,.T.);
#14199=EDGE_CURVE('',#11561,#11654,#1865,.T.);
#14200=EDGE_CURVE('',#11654,#11654,#10286,.T.);
#14201=EDGE_CURVE('',#11583,#11655,#1866,.T.);
#14202=EDGE_CURVE('',#11655,#11655,#10287,.T.);
#14203=EDGE_CURVE('',#11646,#11656,#1867,.T.);
#14204=EDGE_CURVE('',#11656,#11656,#10288,.T.);
#14205=EDGE_CURVE('',#11613,#11657,#1868,.T.);
#14206=EDGE_CURVE('',#11657,#11607,#1869,.T.);
#14207=EDGE_CURVE('',#11481,#11658,#1870,.T.);
#14208=EDGE_CURVE('',#11658,#11658,#10289,.T.);
#14209=EDGE_CURVE('',#11482,#11659,#1871,.T.);
#14210=EDGE_CURVE('',#11659,#11659,#10290,.T.);
#14211=EDGE_CURVE('',#11483,#11660,#1872,.T.);
#14212=EDGE_CURVE('',#11660,#11660,#10291,.T.);
#14213=EDGE_CURVE('',#11484,#11661,#1873,.T.);
#14214=EDGE_CURVE('',#11661,#11661,#10292,.T.);
#14215=EDGE_CURVE('',#11487,#11662,#1874,.T.);
#14216=EDGE_CURVE('',#11662,#11662,#10293,.T.);
#14217=EDGE_CURVE('',#11488,#11663,#1875,.T.);
#14218=EDGE_CURVE('',#11663,#11663,#10294,.T.);
#14219=EDGE_CURVE('',#11489,#11664,#1876,.T.);
#14220=EDGE_CURVE('',#11664,#11664,#10295,.T.);
#14221=EDGE_CURVE('',#11490,#11665,#1877,.T.);
#14222=EDGE_CURVE('',#11665,#11665,#10296,.T.);
#14223=EDGE_CURVE('',#11491,#11666,#1878,.T.);
#14224=EDGE_CURVE('',#11666,#11666,#10297,.T.);
#14225=EDGE_CURVE('',#11492,#11667,#1879,.T.);
#14226=EDGE_CURVE('',#11667,#11667,#10298,.T.);
#14227=EDGE_CURVE('',#11493,#11668,#1880,.T.);
#14228=EDGE_CURVE('',#11668,#11668,#10299,.T.);
#14229=EDGE_CURVE('',#11494,#11669,#1881,.T.);
#14230=EDGE_CURVE('',#11669,#11669,#10300,.T.);
#14231=EDGE_CURVE('',#11670,#11670,#10301,.T.);
#14232=EDGE_CURVE('',#11670,#11485,#1882,.T.);
#14233=EDGE_CURVE('',#11643,#11576,#1883,.T.);
#14234=EDGE_CURVE('',#11644,#11574,#1884,.T.);
#14235=EDGE_CURVE('',#11645,#11572,#1885,.T.);
#14236=EDGE_CURVE('',#11640,#11554,#1886,.T.);
#14237=EDGE_CURVE('',#11641,#11552,#1887,.T.);
#14238=EDGE_CURVE('',#11642,#11550,#1888,.T.);
#14239=EDGE_CURVE('',#11530,#11470,#1889,.T.);
#14240=EDGE_CURVE('',#11531,#11471,#1890,.T.);
#14241=EDGE_CURVE('',#11532,#11477,#1891,.T.);
#14242=EDGE_CURVE('',#11533,#11476,#1892,.T.);
#14243=EDGE_CURVE('',#11534,#11475,#1893,.T.);
#14244=EDGE_CURVE('',#11535,#11474,#1894,.T.);
#14245=EDGE_CURVE('',#11536,#11473,#1895,.T.);
#14246=EDGE_CURVE('',#11537,#11472,#1896,.T.);
#14247=EDGE_CURVE('',#11462,#11671,#1897,.T.);
#14248=EDGE_CURVE('',#11657,#11671,#10302,.T.);
#14249=EDGE_CURVE('',#11671,#11635,#1898,.T.);
#17802=ORIENTED_EDGE('',*,*,#13905,.T.);
#17803=ORIENTED_EDGE('',*,*,#13906,.T.);
#17804=ORIENTED_EDGE('',*,*,#13907,.T.);
#17805=ORIENTED_EDGE('',*,*,#13908,.T.);
#17806=ORIENTED_EDGE('',*,*,#13907,.F.);
#17807=ORIENTED_EDGE('',*,*,#13909,.T.);
#17808=ORIENTED_EDGE('',*,*,#13910,.T.);
#17809=ORIENTED_EDGE('',*,*,#13911,.F.);
#17810=ORIENTED_EDGE('',*,*,#13906,.F.);
#17811=ORIENTED_EDGE('',*,*,#13912,.T.);
#17812=ORIENTED_EDGE('',*,*,#13913,.F.);
#17813=ORIENTED_EDGE('',*,*,#13914,.F.);
#17814=ORIENTED_EDGE('',*,*,#13915,.T.);
#17815=ORIENTED_EDGE('',*,*,#13916,.T.);
#17816=ORIENTED_EDGE('',*,*,#13917,.T.);
#17817=ORIENTED_EDGE('',*,*,#13918,.T.);
#17818=ORIENTED_EDGE('',*,*,#13919,.T.);
#17819=ORIENTED_EDGE('',*,*,#13920,.T.);
#17820=ORIENTED_EDGE('',*,*,#13921,.T.);
#17821=ORIENTED_EDGE('',*,*,#13922,.F.);
#17822=ORIENTED_EDGE('',*,*,#13923,.F.);
#17823=ORIENTED_EDGE('',*,*,#13924,.T.);
#17824=ORIENTED_EDGE('',*,*,#13925,.F.);
#17825=ORIENTED_EDGE('',*,*,#13909,.F.);
#17826=ORIENTED_EDGE('',*,*,#13908,.F.);
#17827=ORIENTED_EDGE('',*,*,#13926,.T.);
#17828=ORIENTED_EDGE('',*,*,#13927,.T.);
#17829=ORIENTED_EDGE('',*,*,#13928,.T.);
#17830=ORIENTED_EDGE('',*,*,#13929,.T.);
#17831=ORIENTED_EDGE('',*,*,#13930,.T.);
#17832=ORIENTED_EDGE('',*,*,#13914,.T.);
#17833=ORIENTED_EDGE('',*,*,#13931,.T.);
#17834=ORIENTED_EDGE('',*,*,#13932,.T.);
#17835=ORIENTED_EDGE('',*,*,#13931,.F.);
#17836=ORIENTED_EDGE('',*,*,#13913,.T.);
#17837=ORIENTED_EDGE('',*,*,#13933,.T.);
#17838=ORIENTED_EDGE('',*,*,#13922,.T.);
#17839=ORIENTED_EDGE('',*,*,#13934,.T.);
#17840=ORIENTED_EDGE('',*,*,#13932,.F.);
#17841=ORIENTED_EDGE('',*,*,#13935,.T.);
#17842=ORIENTED_EDGE('',*,*,#13936,.T.);
#17843=ORIENTED_EDGE('',*,*,#13937,.T.);
#17844=ORIENTED_EDGE('',*,*,#13938,.T.);
#17845=ORIENTED_EDGE('',*,*,#13939,.T.);
#17846=ORIENTED_EDGE('',*,*,#13940,.T.);
#17847=ORIENTED_EDGE('',*,*,#13941,.T.);
#17848=ORIENTED_EDGE('',*,*,#13942,.T.);
#17849=ORIENTED_EDGE('',*,*,#13943,.F.);
#17850=ORIENTED_EDGE('',*,*,#13944,.T.);
#17851=ORIENTED_EDGE('',*,*,#13945,.T.);
#17852=ORIENTED_EDGE('',*,*,#13946,.T.);
#17853=ORIENTED_EDGE('',*,*,#13947,.T.);
#17854=ORIENTED_EDGE('',*,*,#13948,.T.);
#17855=ORIENTED_EDGE('',*,*,#13949,.T.);
#17856=ORIENTED_EDGE('',*,*,#13946,.F.);
#17857=ORIENTED_EDGE('',*,*,#13950,.T.);
#17858=ORIENTED_EDGE('',*,*,#13951,.T.);
#17859=ORIENTED_EDGE('',*,*,#13952,.T.);
#17860=ORIENTED_EDGE('',*,*,#13948,.F.);
#17861=ORIENTED_EDGE('',*,*,#13953,.T.);
#17862=ORIENTED_EDGE('',*,*,#13954,.T.);
#17863=ORIENTED_EDGE('',*,*,#13955,.T.);
#17864=ORIENTED_EDGE('',*,*,#13951,.F.);
#17865=ORIENTED_EDGE('',*,*,#13956,.T.);
#17866=ORIENTED_EDGE('',*,*,#13957,.T.);
#17867=ORIENTED_EDGE('',*,*,#13958,.T.);
#17868=ORIENTED_EDGE('',*,*,#13954,.F.);
#17869=ORIENTED_EDGE('',*,*,#13959,.T.);
#17870=ORIENTED_EDGE('',*,*,#13960,.T.);
#17871=ORIENTED_EDGE('',*,*,#13961,.T.);
#17872=ORIENTED_EDGE('',*,*,#13957,.F.);
#17873=ORIENTED_EDGE('',*,*,#13962,.T.);
#17874=ORIENTED_EDGE('',*,*,#13963,.T.);
#17875=ORIENTED_EDGE('',*,*,#13964,.T.);
#17876=ORIENTED_EDGE('',*,*,#13960,.F.);
#17877=ORIENTED_EDGE('',*,*,#13965,.T.);
#17878=ORIENTED_EDGE('',*,*,#13944,.F.);
#17879=ORIENTED_EDGE('',*,*,#13966,.T.);
#17880=ORIENTED_EDGE('',*,*,#13963,.F.);
#17881=ORIENTED_EDGE('',*,*,#13967,.T.);
#17882=ORIENTED_EDGE('',*,*,#13961,.F.);
#17883=ORIENTED_EDGE('',*,*,#13968,.T.);
#17884=ORIENTED_EDGE('',*,*,#13969,.F.);
#17885=ORIENTED_EDGE('',*,*,#13970,.F.);
#17886=ORIENTED_EDGE('',*,*,#13964,.F.);
#17887=ORIENTED_EDGE('',*,*,#13971,.T.);
#17888=ORIENTED_EDGE('',*,*,#13972,.F.);
#17889=ORIENTED_EDGE('',*,*,#13968,.F.);
#17890=ORIENTED_EDGE('',*,*,#13966,.F.);
#17891=ORIENTED_EDGE('',*,*,#13973,.T.);
#17892=ORIENTED_EDGE('',*,*,#13974,.F.);
#17893=ORIENTED_EDGE('',*,*,#13971,.F.);
#17894=ORIENTED_EDGE('',*,*,#13947,.F.);
#17895=ORIENTED_EDGE('',*,*,#13975,.T.);
#17896=ORIENTED_EDGE('',*,*,#13976,.F.);
#17897=ORIENTED_EDGE('',*,*,#13973,.F.);
#17898=ORIENTED_EDGE('',*,*,#13945,.F.);
#17899=ORIENTED_EDGE('',*,*,#13967,.F.);
#17900=ORIENTED_EDGE('',*,*,#13965,.F.);
#17901=ORIENTED_EDGE('',*,*,#13962,.F.);
#17902=ORIENTED_EDGE('',*,*,#13959,.F.);
#17903=ORIENTED_EDGE('',*,*,#13956,.F.);
#17904=ORIENTED_EDGE('',*,*,#13953,.F.);
#17905=ORIENTED_EDGE('',*,*,#13950,.F.);
#17906=ORIENTED_EDGE('',*,*,#13977,.T.);
#17907=ORIENTED_EDGE('',*,*,#13978,.T.);
#17908=ORIENTED_EDGE('',*,*,#13979,.T.);
#17909=ORIENTED_EDGE('',*,*,#13980,.T.);
#17910=ORIENTED_EDGE('',*,*,#13981,.T.);
#17911=ORIENTED_EDGE('',*,*,#13982,.T.);
#17912=ORIENTED_EDGE('',*,*,#13983,.T.);
#17913=ORIENTED_EDGE('',*,*,#13984,.T.);
#17914=ORIENTED_EDGE('',*,*,#13981,.F.);
#17915=ORIENTED_EDGE('',*,*,#13985,.T.);
#17916=ORIENTED_EDGE('',*,*,#13986,.T.);
#17917=ORIENTED_EDGE('',*,*,#13987,.T.);
#17918=ORIENTED_EDGE('',*,*,#13983,.F.);
#17919=ORIENTED_EDGE('',*,*,#13988,.T.);
#17920=ORIENTED_EDGE('',*,*,#13989,.T.);
#17921=ORIENTED_EDGE('',*,*,#13990,.T.);
#17922=ORIENTED_EDGE('',*,*,#13986,.F.);
#17923=ORIENTED_EDGE('',*,*,#13969,.T.);
#17924=ORIENTED_EDGE('',*,*,#13991,.T.);
#17925=ORIENTED_EDGE('',*,*,#13992,.T.);
#17926=ORIENTED_EDGE('',*,*,#13989,.F.);
#17927=ORIENTED_EDGE('',*,*,#13972,.T.);
#17928=ORIENTED_EDGE('',*,*,#13993,.T.);
#17929=ORIENTED_EDGE('',*,*,#13994,.T.);
#17930=ORIENTED_EDGE('',*,*,#13991,.F.);
#17931=ORIENTED_EDGE('',*,*,#13974,.T.);
#17932=ORIENTED_EDGE('',*,*,#13995,.T.);
#17933=ORIENTED_EDGE('',*,*,#13996,.T.);
#17934=ORIENTED_EDGE('',*,*,#13993,.F.);
#17935=ORIENTED_EDGE('',*,*,#13976,.T.);
#17936=ORIENTED_EDGE('',*,*,#13979,.F.);
#17937=ORIENTED_EDGE('',*,*,#13997,.T.);
#17938=ORIENTED_EDGE('',*,*,#13995,.F.);
#17939=ORIENTED_EDGE('',*,*,#13998,.T.);
#17940=ORIENTED_EDGE('',*,*,#13958,.F.);
#17941=ORIENTED_EDGE('',*,*,#13970,.T.);
#17942=ORIENTED_EDGE('',*,*,#13988,.F.);
#17943=ORIENTED_EDGE('',*,*,#13999,.F.);
#17944=ORIENTED_EDGE('',*,*,#13955,.F.);
#17945=ORIENTED_EDGE('',*,*,#13999,.T.);
#17946=ORIENTED_EDGE('',*,*,#13985,.F.);
#17947=ORIENTED_EDGE('',*,*,#14000,.F.);
#17948=ORIENTED_EDGE('',*,*,#13952,.F.);
#17949=ORIENTED_EDGE('',*,*,#14000,.T.);
#17950=ORIENTED_EDGE('',*,*,#13980,.F.);
#17951=ORIENTED_EDGE('',*,*,#14001,.F.);
#17952=ORIENTED_EDGE('',*,*,#13982,.F.);
#17953=ORIENTED_EDGE('',*,*,#13984,.F.);
#17954=ORIENTED_EDGE('',*,*,#13987,.F.);
#17955=ORIENTED_EDGE('',*,*,#13990,.F.);
#17956=ORIENTED_EDGE('',*,*,#13992,.F.);
#17957=ORIENTED_EDGE('',*,*,#13994,.F.);
#17958=ORIENTED_EDGE('',*,*,#13996,.F.);
#17959=ORIENTED_EDGE('',*,*,#13997,.F.);
#17960=ORIENTED_EDGE('',*,*,#14002,.F.);
#17961=ORIENTED_EDGE('',*,*,#14003,.F.);
#17962=ORIENTED_EDGE('',*,*,#14004,.F.);
#17963=ORIENTED_EDGE('',*,*,#14005,.F.);
#17964=ORIENTED_EDGE('',*,*,#14006,.F.);
#17965=ORIENTED_EDGE('',*,*,#14007,.F.);
#17966=ORIENTED_EDGE('',*,*,#14008,.F.);
#17967=ORIENTED_EDGE('',*,*,#14009,.F.);
#17968=ORIENTED_EDGE('',*,*,#14010,.T.);
#17969=ORIENTED_EDGE('',*,*,#14011,.T.);
#17970=ORIENTED_EDGE('',*,*,#14012,.T.);
#17971=ORIENTED_EDGE('',*,*,#14013,.T.);
#17972=ORIENTED_EDGE('',*,*,#14014,.T.);
#17973=ORIENTED_EDGE('',*,*,#14015,.T.);
#17974=ORIENTED_EDGE('',*,*,#14016,.T.);
#17975=ORIENTED_EDGE('',*,*,#14017,.T.);
#17976=ORIENTED_EDGE('',*,*,#14014,.F.);
#17977=ORIENTED_EDGE('',*,*,#14018,.T.);
#17978=ORIENTED_EDGE('',*,*,#14019,.T.);
#17979=ORIENTED_EDGE('',*,*,#14020,.T.);
#17980=ORIENTED_EDGE('',*,*,#14016,.F.);
#17981=ORIENTED_EDGE('',*,*,#14021,.T.);
#17982=ORIENTED_EDGE('',*,*,#14022,.T.);
#17983=ORIENTED_EDGE('',*,*,#14023,.T.);
#17984=ORIENTED_EDGE('',*,*,#14019,.F.);
#17985=ORIENTED_EDGE('',*,*,#14024,.T.);
#17986=ORIENTED_EDGE('',*,*,#14025,.T.);
#17987=ORIENTED_EDGE('',*,*,#14026,.T.);
#17988=ORIENTED_EDGE('',*,*,#14022,.F.);
#17989=ORIENTED_EDGE('',*,*,#14027,.T.);
#17990=ORIENTED_EDGE('',*,*,#14028,.T.);
#17991=ORIENTED_EDGE('',*,*,#14029,.T.);
#17992=ORIENTED_EDGE('',*,*,#14025,.F.);
#17993=ORIENTED_EDGE('',*,*,#14030,.T.);
#17994=ORIENTED_EDGE('',*,*,#14031,.T.);
#17995=ORIENTED_EDGE('',*,*,#14032,.T.);
#17996=ORIENTED_EDGE('',*,*,#14028,.F.);
#17997=ORIENTED_EDGE('',*,*,#14033,.T.);
#17998=ORIENTED_EDGE('',*,*,#14012,.F.);
#17999=ORIENTED_EDGE('',*,*,#14034,.T.);
#18000=ORIENTED_EDGE('',*,*,#14031,.F.);
#18001=ORIENTED_EDGE('',*,*,#14035,.T.);
#18002=ORIENTED_EDGE('',*,*,#14024,.F.);
#18003=ORIENTED_EDGE('',*,*,#14036,.F.);
#18004=ORIENTED_EDGE('',*,*,#14037,.F.);
#18005=ORIENTED_EDGE('',*,*,#14038,.T.);
#18006=ORIENTED_EDGE('',*,*,#14021,.F.);
#18007=ORIENTED_EDGE('',*,*,#14039,.F.);
#18008=ORIENTED_EDGE('',*,*,#14040,.F.);
#18009=ORIENTED_EDGE('',*,*,#14036,.T.);
#18010=ORIENTED_EDGE('',*,*,#14018,.F.);
#18011=ORIENTED_EDGE('',*,*,#14041,.F.);
#18012=ORIENTED_EDGE('',*,*,#14042,.F.);
#18013=ORIENTED_EDGE('',*,*,#14039,.T.);
#18014=ORIENTED_EDGE('',*,*,#14013,.F.);
#18015=ORIENTED_EDGE('',*,*,#14043,.F.);
#18016=ORIENTED_EDGE('',*,*,#14044,.F.);
#18017=ORIENTED_EDGE('',*,*,#14041,.T.);
#18018=ORIENTED_EDGE('',*,*,#14015,.F.);
#18019=ORIENTED_EDGE('',*,*,#14017,.F.);
#18020=ORIENTED_EDGE('',*,*,#14020,.F.);
#18021=ORIENTED_EDGE('',*,*,#14023,.F.);
#18022=ORIENTED_EDGE('',*,*,#14026,.F.);
#18023=ORIENTED_EDGE('',*,*,#14029,.F.);
#18024=ORIENTED_EDGE('',*,*,#14032,.F.);
#18025=ORIENTED_EDGE('',*,*,#14034,.F.);
#18026=ORIENTED_EDGE('',*,*,#14045,.T.);
#18027=ORIENTED_EDGE('',*,*,#14046,.T.);
#18028=ORIENTED_EDGE('',*,*,#14047,.T.);
#18029=ORIENTED_EDGE('',*,*,#14048,.T.);
#18030=ORIENTED_EDGE('',*,*,#14049,.T.);
#18031=ORIENTED_EDGE('',*,*,#14050,.T.);
#18032=ORIENTED_EDGE('',*,*,#14051,.T.);
#18033=ORIENTED_EDGE('',*,*,#14048,.F.);
#18034=ORIENTED_EDGE('',*,*,#14052,.T.);
#18035=ORIENTED_EDGE('',*,*,#14053,.T.);
#18036=ORIENTED_EDGE('',*,*,#14054,.T.);
#18037=ORIENTED_EDGE('',*,*,#14050,.F.);
#18038=ORIENTED_EDGE('',*,*,#14055,.T.);
#18039=ORIENTED_EDGE('',*,*,#14056,.T.);
#18040=ORIENTED_EDGE('',*,*,#14057,.T.);
#18041=ORIENTED_EDGE('',*,*,#14053,.F.);
#18042=ORIENTED_EDGE('',*,*,#14058,.T.);
#18043=ORIENTED_EDGE('',*,*,#14059,.T.);
#18044=ORIENTED_EDGE('',*,*,#14060,.T.);
#18045=ORIENTED_EDGE('',*,*,#14056,.F.);
#18046=ORIENTED_EDGE('',*,*,#14061,.T.);
#18047=ORIENTED_EDGE('',*,*,#14062,.T.);
#18048=ORIENTED_EDGE('',*,*,#14063,.T.);
#18049=ORIENTED_EDGE('',*,*,#14059,.F.);
#18050=ORIENTED_EDGE('',*,*,#14064,.T.);
#18051=ORIENTED_EDGE('',*,*,#14065,.T.);
#18052=ORIENTED_EDGE('',*,*,#14066,.T.);
#18053=ORIENTED_EDGE('',*,*,#14062,.F.);
#18054=ORIENTED_EDGE('',*,*,#14067,.T.);
#18055=ORIENTED_EDGE('',*,*,#14046,.F.);
#18056=ORIENTED_EDGE('',*,*,#14068,.T.);
#18057=ORIENTED_EDGE('',*,*,#14065,.F.);
#18058=ORIENTED_EDGE('',*,*,#14069,.T.);
#18059=ORIENTED_EDGE('',*,*,#14058,.F.);
#18060=ORIENTED_EDGE('',*,*,#14070,.F.);
#18061=ORIENTED_EDGE('',*,*,#14071,.F.);
#18062=ORIENTED_EDGE('',*,*,#14072,.T.);
#18063=ORIENTED_EDGE('',*,*,#14055,.F.);
#18064=ORIENTED_EDGE('',*,*,#14073,.F.);
#18065=ORIENTED_EDGE('',*,*,#14074,.F.);
#18066=ORIENTED_EDGE('',*,*,#14070,.T.);
#18067=ORIENTED_EDGE('',*,*,#14052,.F.);
#18068=ORIENTED_EDGE('',*,*,#14075,.F.);
#18069=ORIENTED_EDGE('',*,*,#14076,.F.);
#18070=ORIENTED_EDGE('',*,*,#14073,.T.);
#18071=ORIENTED_EDGE('',*,*,#14047,.F.);
#18072=ORIENTED_EDGE('',*,*,#14077,.F.);
#18073=ORIENTED_EDGE('',*,*,#14078,.F.);
#18074=ORIENTED_EDGE('',*,*,#14075,.T.);
#18075=ORIENTED_EDGE('',*,*,#14049,.F.);
#18076=ORIENTED_EDGE('',*,*,#14051,.F.);
#18077=ORIENTED_EDGE('',*,*,#14054,.F.);
#18078=ORIENTED_EDGE('',*,*,#14057,.F.);
#18079=ORIENTED_EDGE('',*,*,#14060,.F.);
#18080=ORIENTED_EDGE('',*,*,#14063,.F.);
#18081=ORIENTED_EDGE('',*,*,#14066,.F.);
#18082=ORIENTED_EDGE('',*,*,#14068,.F.);
#18083=ORIENTED_EDGE('',*,*,#14079,.T.);
#18084=ORIENTED_EDGE('',*,*,#13943,.T.);
#18085=ORIENTED_EDGE('',*,*,#14080,.T.);
#18086=ORIENTED_EDGE('',*,*,#14081,.T.);
#18087=ORIENTED_EDGE('',*,*,#14080,.F.);
#18088=ORIENTED_EDGE('',*,*,#14081,.F.);
#18089=ORIENTED_EDGE('',*,*,#14082,.T.);
#18090=ORIENTED_EDGE('',*,*,#14083,.T.);
#18091=ORIENTED_EDGE('',*,*,#14084,.F.);
#18092=ORIENTED_EDGE('',*,*,#14085,.F.);
#18093=ORIENTED_EDGE('',*,*,#14086,.T.);
#18094=ORIENTED_EDGE('',*,*,#14087,.F.);
#18095=ORIENTED_EDGE('',*,*,#14088,.T.);
#18096=ORIENTED_EDGE('',*,*,#14089,.T.);
#18097=ORIENTED_EDGE('',*,*,#14082,.F.);
#18098=ORIENTED_EDGE('',*,*,#14090,.T.);
#18099=ORIENTED_EDGE('',*,*,#14091,.T.);
#18100=ORIENTED_EDGE('',*,*,#14092,.T.);
#18101=ORIENTED_EDGE('',*,*,#14091,.F.);
#18102=ORIENTED_EDGE('',*,*,#14093,.F.);
#18103=ORIENTED_EDGE('',*,*,#14086,.F.);
#18104=ORIENTED_EDGE('',*,*,#14094,.F.);
#18105=ORIENTED_EDGE('',*,*,#14095,.F.);
#18106=ORIENTED_EDGE('',*,*,#14090,.F.);
#18107=ORIENTED_EDGE('',*,*,#14092,.F.);
#18108=ORIENTED_EDGE('',*,*,#14096,.T.);
#18109=ORIENTED_EDGE('',*,*,#14097,.T.);
#18110=ORIENTED_EDGE('',*,*,#14096,.F.);
#18111=ORIENTED_EDGE('',*,*,#14098,.T.);
#18112=ORIENTED_EDGE('',*,*,#14087,.T.);
#18113=ORIENTED_EDGE('',*,*,#14093,.T.);
#18114=ORIENTED_EDGE('',*,*,#14099,.T.);
#18115=ORIENTED_EDGE('',*,*,#14100,.T.);
#18116=ORIENTED_EDGE('',*,*,#14099,.F.);
#18117=ORIENTED_EDGE('',*,*,#14095,.T.);
#18118=ORIENTED_EDGE('',*,*,#14101,.T.);
#18119=ORIENTED_EDGE('',*,*,#14094,.T.);
#18120=ORIENTED_EDGE('',*,*,#14085,.T.);
#18121=ORIENTED_EDGE('',*,*,#14102,.T.);
#18122=ORIENTED_EDGE('',*,*,#14101,.F.);
#18123=ORIENTED_EDGE('',*,*,#14098,.F.);
#18124=ORIENTED_EDGE('',*,*,#14103,.T.);
#18125=ORIENTED_EDGE('',*,*,#14104,.T.);
#18126=ORIENTED_EDGE('',*,*,#14088,.F.);
#18127=ORIENTED_EDGE('',*,*,#14100,.F.);
#18128=ORIENTED_EDGE('',*,*,#14105,.T.);
#18129=ORIENTED_EDGE('',*,*,#14106,.T.);
#18130=ORIENTED_EDGE('',*,*,#14103,.F.);
#18131=ORIENTED_EDGE('',*,*,#14102,.F.);
#18132=ORIENTED_EDGE('',*,*,#14084,.T.);
#18133=ORIENTED_EDGE('',*,*,#14107,.T.);
#18134=ORIENTED_EDGE('',*,*,#14105,.F.);
#18135=ORIENTED_EDGE('',*,*,#14108,.T.);
#18136=ORIENTED_EDGE('',*,*,#14109,.T.);
#18137=ORIENTED_EDGE('',*,*,#14110,.T.);
#18138=ORIENTED_EDGE('',*,*,#14111,.T.);
#18139=ORIENTED_EDGE('',*,*,#14112,.T.);
#18140=ORIENTED_EDGE('',*,*,#14113,.T.);
#18141=ORIENTED_EDGE('',*,*,#14114,.T.);
#18142=ORIENTED_EDGE('',*,*,#14111,.F.);
#18143=ORIENTED_EDGE('',*,*,#14115,.T.);
#18144=ORIENTED_EDGE('',*,*,#14116,.T.);
#18145=ORIENTED_EDGE('',*,*,#14117,.T.);
#18146=ORIENTED_EDGE('',*,*,#14113,.F.);
#18147=ORIENTED_EDGE('',*,*,#14118,.T.);
#18148=ORIENTED_EDGE('',*,*,#14108,.F.);
#18149=ORIENTED_EDGE('',*,*,#14119,.T.);
#18150=ORIENTED_EDGE('',*,*,#14116,.F.);
#18151=ORIENTED_EDGE('',*,*,#14120,.T.);
#18152=ORIENTED_EDGE('',*,*,#14119,.F.);
#18153=ORIENTED_EDGE('',*,*,#14121,.T.);
#18154=ORIENTED_EDGE('',*,*,#14122,.F.);
#18155=ORIENTED_EDGE('',*,*,#14123,.F.);
#18156=ORIENTED_EDGE('',*,*,#14124,.T.);
#18157=ORIENTED_EDGE('',*,*,#14125,.T.);
#18158=ORIENTED_EDGE('',*,*,#14112,.F.);
#18159=ORIENTED_EDGE('',*,*,#14126,.T.);
#18160=ORIENTED_EDGE('',*,*,#14127,.F.);
#18161=ORIENTED_EDGE('',*,*,#14121,.F.);
#18162=ORIENTED_EDGE('',*,*,#14109,.F.);
#18163=ORIENTED_EDGE('',*,*,#14120,.F.);
#18164=ORIENTED_EDGE('',*,*,#14118,.F.);
#18165=ORIENTED_EDGE('',*,*,#14115,.F.);
#18166=ORIENTED_EDGE('',*,*,#14110,.F.);
#18167=ORIENTED_EDGE('',*,*,#14128,.T.);
#18168=ORIENTED_EDGE('',*,*,#14129,.T.);
#18169=ORIENTED_EDGE('',*,*,#14128,.F.);
#18170=ORIENTED_EDGE('',*,*,#13925,.T.);
#18171=ORIENTED_EDGE('',*,*,#14130,.T.);
#18172=ORIENTED_EDGE('',*,*,#14131,.T.);
#18173=ORIENTED_EDGE('',*,*,#14132,.T.);
#18174=ORIENTED_EDGE('',*,*,#13910,.F.);
#18175=ORIENTED_EDGE('',*,*,#14133,.T.);
#18176=ORIENTED_EDGE('',*,*,#14134,.T.);
#18177=ORIENTED_EDGE('',*,*,#14135,.T.);
#18178=ORIENTED_EDGE('',*,*,#14136,.T.);
#18179=ORIENTED_EDGE('',*,*,#14137,.T.);
#18180=ORIENTED_EDGE('',*,*,#14138,.T.);
#18181=ORIENTED_EDGE('',*,*,#14135,.F.);
#18182=ORIENTED_EDGE('',*,*,#14139,.T.);
#18183=ORIENTED_EDGE('',*,*,#13923,.T.);
#18184=ORIENTED_EDGE('',*,*,#14140,.T.);
#18185=ORIENTED_EDGE('',*,*,#14137,.F.);
#18186=ORIENTED_EDGE('',*,*,#14141,.T.);
#18187=ORIENTED_EDGE('',*,*,#14133,.F.);
#18188=ORIENTED_EDGE('',*,*,#14142,.T.);
#18189=ORIENTED_EDGE('',*,*,#14131,.F.);
#18190=ORIENTED_EDGE('',*,*,#14143,.T.);
#18191=ORIENTED_EDGE('',*,*,#14138,.F.);
#18192=ORIENTED_EDGE('',*,*,#14144,.T.);
#18193=ORIENTED_EDGE('',*,*,#14145,.F.);
#18194=ORIENTED_EDGE('',*,*,#14146,.F.);
#18195=ORIENTED_EDGE('',*,*,#14147,.F.);
#18196=ORIENTED_EDGE('',*,*,#14148,.F.);
#18197=ORIENTED_EDGE('',*,*,#14140,.F.);
#18198=ORIENTED_EDGE('',*,*,#13933,.F.);
#18199=ORIENTED_EDGE('',*,*,#14149,.T.);
#18200=ORIENTED_EDGE('',*,*,#14123,.T.);
#18201=ORIENTED_EDGE('',*,*,#14150,.F.);
#18202=ORIENTED_EDGE('',*,*,#14144,.F.);
#18203=ORIENTED_EDGE('',*,*,#14141,.F.);
#18204=ORIENTED_EDGE('',*,*,#14139,.F.);
#18205=ORIENTED_EDGE('',*,*,#14134,.F.);
#18206=ORIENTED_EDGE('',*,*,#14143,.F.);
#18207=ORIENTED_EDGE('',*,*,#14130,.F.);
#18208=ORIENTED_EDGE('',*,*,#13924,.F.);
#18209=ORIENTED_EDGE('',*,*,#14151,.T.);
#18210=ORIENTED_EDGE('',*,*,#14152,.T.);
#18211=ORIENTED_EDGE('',*,*,#14153,.T.);
#18212=ORIENTED_EDGE('',*,*,#14154,.T.);
#18213=ORIENTED_EDGE('',*,*,#14155,.T.);
#18214=ORIENTED_EDGE('',*,*,#14156,.T.);
#18215=ORIENTED_EDGE('',*,*,#14153,.F.);
#18216=ORIENTED_EDGE('',*,*,#14145,.T.);
#18217=ORIENTED_EDGE('',*,*,#14157,.T.);
#18218=ORIENTED_EDGE('',*,*,#14158,.T.);
#18219=ORIENTED_EDGE('',*,*,#14155,.F.);
#18220=ORIENTED_EDGE('',*,*,#14150,.T.);
#18221=ORIENTED_EDGE('',*,*,#14159,.T.);
#18222=ORIENTED_EDGE('',*,*,#14160,.T.);
#18223=ORIENTED_EDGE('',*,*,#14157,.F.);
#18224=ORIENTED_EDGE('',*,*,#14122,.T.);
#18225=ORIENTED_EDGE('',*,*,#14161,.T.);
#18226=ORIENTED_EDGE('',*,*,#14162,.T.);
#18227=ORIENTED_EDGE('',*,*,#14159,.F.);
#18228=ORIENTED_EDGE('',*,*,#14127,.T.);
#18229=ORIENTED_EDGE('',*,*,#14163,.T.);
#18230=ORIENTED_EDGE('',*,*,#14164,.T.);
#18231=ORIENTED_EDGE('',*,*,#14161,.F.);
#18232=ORIENTED_EDGE('',*,*,#14165,.T.);
#18233=ORIENTED_EDGE('',*,*,#14166,.T.);
#18234=ORIENTED_EDGE('',*,*,#14167,.T.);
#18235=ORIENTED_EDGE('',*,*,#14163,.F.);
#18236=ORIENTED_EDGE('',*,*,#14168,.T.);
#18237=ORIENTED_EDGE('',*,*,#14151,.F.);
#18238=ORIENTED_EDGE('',*,*,#14169,.T.);
#18239=ORIENTED_EDGE('',*,*,#14166,.F.);
#18240=ORIENTED_EDGE('',*,*,#14170,.T.);
#18241=ORIENTED_EDGE('',*,*,#14152,.F.);
#18242=ORIENTED_EDGE('',*,*,#14171,.F.);
#18243=ORIENTED_EDGE('',*,*,#14172,.F.);
#18244=ORIENTED_EDGE('',*,*,#14146,.T.);
#18245=ORIENTED_EDGE('',*,*,#14154,.F.);
#18246=ORIENTED_EDGE('',*,*,#14156,.F.);
#18247=ORIENTED_EDGE('',*,*,#14158,.F.);
#18248=ORIENTED_EDGE('',*,*,#14160,.F.);
#18249=ORIENTED_EDGE('',*,*,#14162,.F.);
#18250=ORIENTED_EDGE('',*,*,#14164,.F.);
#18251=ORIENTED_EDGE('',*,*,#14167,.F.);
#18252=ORIENTED_EDGE('',*,*,#14169,.F.);
#18253=ORIENTED_EDGE('',*,*,#14044,.T.);
#18254=ORIENTED_EDGE('',*,*,#14173,.T.);
#18255=ORIENTED_EDGE('',*,*,#14174,.T.);
#18256=ORIENTED_EDGE('',*,*,#14175,.T.);
#18257=ORIENTED_EDGE('',*,*,#14176,.T.);
#18258=ORIENTED_EDGE('',*,*,#14037,.T.);
#18259=ORIENTED_EDGE('',*,*,#14040,.T.);
#18260=ORIENTED_EDGE('',*,*,#14042,.T.);
#18261=ORIENTED_EDGE('',*,*,#14078,.T.);
#18262=ORIENTED_EDGE('',*,*,#14177,.T.);
#18263=ORIENTED_EDGE('',*,*,#14178,.T.);
#18264=ORIENTED_EDGE('',*,*,#14179,.T.);
#18265=ORIENTED_EDGE('',*,*,#14180,.T.);
#18266=ORIENTED_EDGE('',*,*,#14071,.T.);
#18267=ORIENTED_EDGE('',*,*,#14074,.T.);
#18268=ORIENTED_EDGE('',*,*,#14076,.T.);
#18269=ORIENTED_EDGE('',*,*,#14181,.T.);
#18270=ORIENTED_EDGE('',*,*,#14182,.T.);
#18271=ORIENTED_EDGE('',*,*,#14183,.T.);
#18272=ORIENTED_EDGE('',*,*,#14184,.T.);
#18273=ORIENTED_EDGE('',*,*,#14185,.T.);
#18274=ORIENTED_EDGE('',*,*,#14172,.T.);
#18275=ORIENTED_EDGE('',*,*,#14186,.T.);
#18276=ORIENTED_EDGE('',*,*,#14147,.T.);
#18277=ORIENTED_EDGE('',*,*,#14185,.F.);
#18278=ORIENTED_EDGE('',*,*,#14187,.T.);
#18279=ORIENTED_EDGE('',*,*,#14188,.T.);
#18280=ORIENTED_EDGE('',*,*,#14189,.T.);
#18281=ORIENTED_EDGE('',*,*,#14186,.F.);
#18282=ORIENTED_EDGE('',*,*,#14190,.T.);
#18283=ORIENTED_EDGE('',*,*,#14182,.F.);
#18284=ORIENTED_EDGE('',*,*,#14191,.T.);
#18285=ORIENTED_EDGE('',*,*,#14188,.F.);
#18286=ORIENTED_EDGE('',*,*,#14192,.T.);
#18287=ORIENTED_EDGE('',*,*,#14142,.F.);
#18288=ORIENTED_EDGE('',*,*,#14193,.T.);
#18289=ORIENTED_EDGE('',*,*,#14191,.F.);
#18290=ORIENTED_EDGE('',*,*,#14171,.T.);
#18291=ORIENTED_EDGE('',*,*,#14170,.F.);
#18292=ORIENTED_EDGE('',*,*,#14194,.F.);
#18293=ORIENTED_EDGE('',*,*,#14183,.F.);
#18294=ORIENTED_EDGE('',*,*,#14192,.F.);
#18295=ORIENTED_EDGE('',*,*,#14190,.F.);
#18296=ORIENTED_EDGE('',*,*,#14187,.F.);
#18297=ORIENTED_EDGE('',*,*,#14184,.F.);
#18298=ORIENTED_EDGE('',*,*,#14195,.T.);
#18299=ORIENTED_EDGE('',*,*,#14196,.T.);
#18300=ORIENTED_EDGE('',*,*,#14195,.F.);
#18301=ORIENTED_EDGE('',*,*,#14011,.F.);
#18302=ORIENTED_EDGE('',*,*,#14197,.T.);
#18303=ORIENTED_EDGE('',*,*,#13978,.F.);
#18304=ORIENTED_EDGE('',*,*,#14197,.F.);
#18305=ORIENTED_EDGE('',*,*,#14010,.F.);
#18306=ORIENTED_EDGE('',*,*,#14198,.T.);
#18307=ORIENTED_EDGE('',*,*,#13977,.F.);
#18308=ORIENTED_EDGE('',*,*,#14198,.F.);
#18309=ORIENTED_EDGE('',*,*,#14045,.F.);
#18310=ORIENTED_EDGE('',*,*,#14199,.T.);
#18311=ORIENTED_EDGE('',*,*,#14200,.T.);
#18312=ORIENTED_EDGE('',*,*,#14199,.F.);
#18313=ORIENTED_EDGE('',*,*,#14200,.F.);
#18314=ORIENTED_EDGE('',*,*,#14079,.F.);
#18315=ORIENTED_EDGE('',*,*,#14201,.T.);
#18316=ORIENTED_EDGE('',*,*,#14202,.T.);
#18317=ORIENTED_EDGE('',*,*,#14201,.F.);
#18318=ORIENTED_EDGE('',*,*,#14202,.F.);
#18319=ORIENTED_EDGE('',*,*,#14181,.F.);
#18320=ORIENTED_EDGE('',*,*,#14203,.T.);
#18321=ORIENTED_EDGE('',*,*,#14204,.T.);
#18322=ORIENTED_EDGE('',*,*,#14203,.F.);
#18323=ORIENTED_EDGE('',*,*,#14204,.F.);
#18324=ORIENTED_EDGE('',*,*,#14196,.F.);
#18325=ORIENTED_EDGE('',*,*,#14136,.F.);
#18326=ORIENTED_EDGE('',*,*,#14148,.T.);
#18327=ORIENTED_EDGE('',*,*,#14189,.F.);
#18328=ORIENTED_EDGE('',*,*,#14193,.F.);
#18329=ORIENTED_EDGE('',*,*,#14129,.F.);
#18330=ORIENTED_EDGE('',*,*,#14117,.F.);
#18331=ORIENTED_EDGE('',*,*,#14125,.F.);
#18332=ORIENTED_EDGE('',*,*,#14205,.T.);
#18333=ORIENTED_EDGE('',*,*,#14206,.T.);
#18334=ORIENTED_EDGE('',*,*,#13926,.F.);
#18335=ORIENTED_EDGE('',*,*,#14207,.T.);
#18336=ORIENTED_EDGE('',*,*,#14208,.T.);
#18337=ORIENTED_EDGE('',*,*,#14207,.F.);
#18338=ORIENTED_EDGE('',*,*,#14208,.F.);
#18339=ORIENTED_EDGE('',*,*,#13927,.F.);
#18340=ORIENTED_EDGE('',*,*,#14209,.T.);
#18341=ORIENTED_EDGE('',*,*,#14210,.T.);
#18342=ORIENTED_EDGE('',*,*,#14209,.F.);
#18343=ORIENTED_EDGE('',*,*,#14210,.F.);
#18344=ORIENTED_EDGE('',*,*,#13928,.F.);
#18345=ORIENTED_EDGE('',*,*,#14211,.T.);
#18346=ORIENTED_EDGE('',*,*,#14212,.T.);
#18347=ORIENTED_EDGE('',*,*,#14211,.F.);
#18348=ORIENTED_EDGE('',*,*,#14212,.F.);
#18349=ORIENTED_EDGE('',*,*,#13929,.F.);
#18350=ORIENTED_EDGE('',*,*,#14213,.T.);
#18351=ORIENTED_EDGE('',*,*,#14214,.T.);
#18352=ORIENTED_EDGE('',*,*,#14213,.F.);
#18353=ORIENTED_EDGE('',*,*,#14214,.F.);
#18354=ORIENTED_EDGE('',*,*,#13935,.F.);
#18355=ORIENTED_EDGE('',*,*,#14215,.T.);
#18356=ORIENTED_EDGE('',*,*,#14216,.T.);
#18357=ORIENTED_EDGE('',*,*,#14215,.F.);
#18358=ORIENTED_EDGE('',*,*,#14216,.F.);
#18359=ORIENTED_EDGE('',*,*,#13936,.F.);
#18360=ORIENTED_EDGE('',*,*,#14217,.T.);
#18361=ORIENTED_EDGE('',*,*,#14218,.T.);
#18362=ORIENTED_EDGE('',*,*,#14217,.F.);
#18363=ORIENTED_EDGE('',*,*,#14218,.F.);
#18364=ORIENTED_EDGE('',*,*,#13937,.F.);
#18365=ORIENTED_EDGE('',*,*,#14219,.T.);
#18366=ORIENTED_EDGE('',*,*,#14220,.T.);
#18367=ORIENTED_EDGE('',*,*,#14219,.F.);
#18368=ORIENTED_EDGE('',*,*,#14220,.F.);
#18369=ORIENTED_EDGE('',*,*,#13938,.F.);
#18370=ORIENTED_EDGE('',*,*,#14221,.T.);
#18371=ORIENTED_EDGE('',*,*,#14222,.T.);
#18372=ORIENTED_EDGE('',*,*,#14221,.F.);
#18373=ORIENTED_EDGE('',*,*,#14222,.F.);
#18374=ORIENTED_EDGE('',*,*,#13939,.F.);
#18375=ORIENTED_EDGE('',*,*,#14223,.T.);
#18376=ORIENTED_EDGE('',*,*,#14224,.T.);
#18377=ORIENTED_EDGE('',*,*,#14223,.F.);
#18378=ORIENTED_EDGE('',*,*,#14224,.F.);
#18379=ORIENTED_EDGE('',*,*,#13940,.F.);
#18380=ORIENTED_EDGE('',*,*,#14225,.T.);
#18381=ORIENTED_EDGE('',*,*,#14226,.T.);
#18382=ORIENTED_EDGE('',*,*,#14225,.F.);
#18383=ORIENTED_EDGE('',*,*,#14226,.F.);
#18384=ORIENTED_EDGE('',*,*,#13941,.F.);
#18385=ORIENTED_EDGE('',*,*,#14227,.T.);
#18386=ORIENTED_EDGE('',*,*,#14228,.T.);
#18387=ORIENTED_EDGE('',*,*,#14227,.F.);
#18388=ORIENTED_EDGE('',*,*,#14228,.F.);
#18389=ORIENTED_EDGE('',*,*,#13942,.F.);
#18390=ORIENTED_EDGE('',*,*,#14229,.T.);
#18391=ORIENTED_EDGE('',*,*,#14230,.T.);
#18392=ORIENTED_EDGE('',*,*,#14229,.F.);
#18393=ORIENTED_EDGE('',*,*,#14230,.F.);
#18394=ORIENTED_EDGE('',*,*,#14107,.F.);
#18395=ORIENTED_EDGE('',*,*,#14083,.F.);
#18396=ORIENTED_EDGE('',*,*,#14089,.F.);
#18397=ORIENTED_EDGE('',*,*,#14104,.F.);
#18398=ORIENTED_EDGE('',*,*,#14106,.F.);
#18399=ORIENTED_EDGE('',*,*,#14097,.F.);
#18400=ORIENTED_EDGE('',*,*,#14231,.T.);
#18401=ORIENTED_EDGE('',*,*,#14231,.F.);
#18402=ORIENTED_EDGE('',*,*,#14232,.T.);
#18403=ORIENTED_EDGE('',*,*,#13930,.F.);
#18404=ORIENTED_EDGE('',*,*,#14232,.F.);
#18405=ORIENTED_EDGE('',*,*,#14069,.F.);
#18406=ORIENTED_EDGE('',*,*,#14233,.F.);
#18407=ORIENTED_EDGE('',*,*,#14177,.F.);
#18408=ORIENTED_EDGE('',*,*,#14077,.T.);
#18409=ORIENTED_EDGE('',*,*,#14067,.F.);
#18410=ORIENTED_EDGE('',*,*,#14234,.F.);
#18411=ORIENTED_EDGE('',*,*,#14178,.F.);
#18412=ORIENTED_EDGE('',*,*,#14233,.T.);
#18413=ORIENTED_EDGE('',*,*,#14064,.F.);
#18414=ORIENTED_EDGE('',*,*,#14235,.F.);
#18415=ORIENTED_EDGE('',*,*,#14179,.F.);
#18416=ORIENTED_EDGE('',*,*,#14234,.T.);
#18417=ORIENTED_EDGE('',*,*,#14061,.F.);
#18418=ORIENTED_EDGE('',*,*,#14072,.F.);
#18419=ORIENTED_EDGE('',*,*,#14180,.F.);
#18420=ORIENTED_EDGE('',*,*,#14235,.T.);
#18421=ORIENTED_EDGE('',*,*,#14035,.F.);
#18422=ORIENTED_EDGE('',*,*,#14236,.F.);
#18423=ORIENTED_EDGE('',*,*,#14173,.F.);
#18424=ORIENTED_EDGE('',*,*,#14043,.T.);
#18425=ORIENTED_EDGE('',*,*,#14033,.F.);
#18426=ORIENTED_EDGE('',*,*,#14237,.F.);
#18427=ORIENTED_EDGE('',*,*,#14174,.F.);
#18428=ORIENTED_EDGE('',*,*,#14236,.T.);
#18429=ORIENTED_EDGE('',*,*,#14030,.F.);
#18430=ORIENTED_EDGE('',*,*,#14238,.F.);
#18431=ORIENTED_EDGE('',*,*,#14175,.F.);
#18432=ORIENTED_EDGE('',*,*,#14237,.T.);
#18433=ORIENTED_EDGE('',*,*,#14027,.F.);
#18434=ORIENTED_EDGE('',*,*,#14038,.F.);
#18435=ORIENTED_EDGE('',*,*,#14176,.F.);
#18436=ORIENTED_EDGE('',*,*,#14238,.T.);
#18437=ORIENTED_EDGE('',*,*,#13949,.F.);
#18438=ORIENTED_EDGE('',*,*,#14001,.T.);
#18439=ORIENTED_EDGE('',*,*,#13998,.F.);
#18440=ORIENTED_EDGE('',*,*,#13975,.F.);
#18441=ORIENTED_EDGE('',*,*,#13915,.F.);
#18442=ORIENTED_EDGE('',*,*,#14239,.F.);
#18443=ORIENTED_EDGE('',*,*,#14002,.T.);
#18444=ORIENTED_EDGE('',*,*,#14240,.T.);
#18445=ORIENTED_EDGE('',*,*,#13934,.F.);
#18446=ORIENTED_EDGE('',*,*,#14241,.F.);
#18447=ORIENTED_EDGE('',*,*,#14003,.T.);
#18448=ORIENTED_EDGE('',*,*,#14239,.T.);
#18449=ORIENTED_EDGE('',*,*,#13921,.F.);
#18450=ORIENTED_EDGE('',*,*,#14242,.F.);
#18451=ORIENTED_EDGE('',*,*,#14004,.T.);
#18452=ORIENTED_EDGE('',*,*,#14241,.T.);
#18453=ORIENTED_EDGE('',*,*,#13920,.F.);
#18454=ORIENTED_EDGE('',*,*,#14243,.F.);
#18455=ORIENTED_EDGE('',*,*,#14005,.T.);
#18456=ORIENTED_EDGE('',*,*,#14242,.T.);
#18457=ORIENTED_EDGE('',*,*,#13919,.F.);
#18458=ORIENTED_EDGE('',*,*,#14244,.F.);
#18459=ORIENTED_EDGE('',*,*,#14006,.T.);
#18460=ORIENTED_EDGE('',*,*,#14243,.T.);
#18461=ORIENTED_EDGE('',*,*,#13918,.F.);
#18462=ORIENTED_EDGE('',*,*,#14245,.F.);
#18463=ORIENTED_EDGE('',*,*,#14007,.T.);
#18464=ORIENTED_EDGE('',*,*,#14244,.T.);
#18465=ORIENTED_EDGE('',*,*,#13917,.F.);
#18466=ORIENTED_EDGE('',*,*,#14246,.F.);
#18467=ORIENTED_EDGE('',*,*,#14008,.T.);
#18468=ORIENTED_EDGE('',*,*,#14245,.T.);
#18469=ORIENTED_EDGE('',*,*,#13916,.F.);
#18470=ORIENTED_EDGE('',*,*,#14240,.F.);
#18471=ORIENTED_EDGE('',*,*,#14009,.T.);
#18472=ORIENTED_EDGE('',*,*,#14246,.T.);
#18473=ORIENTED_EDGE('',*,*,#14247,.T.);
#18474=ORIENTED_EDGE('',*,*,#14248,.F.);
#18475=ORIENTED_EDGE('',*,*,#14205,.F.);
#18476=ORIENTED_EDGE('',*,*,#14124,.F.);
#18477=ORIENTED_EDGE('',*,*,#14149,.F.);
#18478=ORIENTED_EDGE('',*,*,#13912,.F.);
#18479=ORIENTED_EDGE('',*,*,#13905,.F.);
#18480=ORIENTED_EDGE('',*,*,#14132,.F.);
#18481=ORIENTED_EDGE('',*,*,#14194,.T.);
#18482=ORIENTED_EDGE('',*,*,#14168,.F.);
#18483=ORIENTED_EDGE('',*,*,#14249,.F.);
#18484=ORIENTED_EDGE('',*,*,#14247,.F.);
#18485=ORIENTED_EDGE('',*,*,#13911,.T.);
#18486=ORIENTED_EDGE('',*,*,#14114,.F.);
#18487=ORIENTED_EDGE('',*,*,#14206,.F.);
#18488=ORIENTED_EDGE('',*,*,#14248,.T.);
#18489=ORIENTED_EDGE('',*,*,#14249,.T.);
#18490=ORIENTED_EDGE('',*,*,#14165,.F.);
#18491=ORIENTED_EDGE('',*,*,#14126,.F.);
#25596=TOROIDAL_SURFACE('',#27464,90.,2.);
#25597=TOROIDAL_SURFACE('',#27481,90.,2.);
#25598=TOROIDAL_SURFACE('',#27609,72.2,2.);
#25599=TOROIDAL_SURFACE('',#27616,22.05,2.);
#25600=TOROIDAL_SURFACE('',#27625,55.,2.);
#25601=TOROIDAL_SURFACE('',#27632,18.75,2.);
#25602=TOROIDAL_SURFACE('',#27639,18.75,2.);
#25603=TOROIDAL_SURFACE('',#27654,3.99999999999996,2.);
#25604=TOROIDAL_SURFACE('',#27659,3.99999999999999,2.);
#25605=TOROIDAL_SURFACE('',#27669,3.99999999999996,2.);
#25606=TOROIDAL_SURFACE('',#27674,3.99999999999997,2.);
#25607=TOROIDAL_SURFACE('',#27679,3.99999999999998,2.);
#25608=TOROIDAL_SURFACE('',#27685,3.99999999999999,2.);
#25609=TOROIDAL_SURFACE('',#27696,18.75,2.);
#25610=TOROIDAL_SURFACE('',#27702,18.75,2.);
#25651=ADVANCED_FACE('',(#6827),#25596,.T.);
#25652=ADVANCED_FACE('',(#6828),#6500,.T.);
#25653=ADVANCED_FACE('',(#6829,#605,#606,#607,#608,#609),#757,.T.);
#25654=ADVANCED_FACE('',(#6830),#25597,.T.);
#25655=ADVANCED_FACE('',(#6831,#610,#611,#612,#613,#614,#615,#616,#617,
#618),#758,.T.);
#25656=ADVANCED_FACE('',(#6832),#6501,.T.);
#25657=ADVANCED_FACE('',(#6833),#584,.F.);
#25658=ADVANCED_FACE('',(#6834),#6502,.T.);
#25659=ADVANCED_FACE('',(#6835),#585,.F.);
#25660=ADVANCED_FACE('',(#6836),#6503,.T.);
#25661=ADVANCED_FACE('',(#6837),#586,.F.);
#25662=ADVANCED_FACE('',(#6838),#6504,.T.);
#25663=ADVANCED_FACE('',(#6839),#587,.F.);
#25664=ADVANCED_FACE('',(#6840),#6505,.T.);
#25665=ADVANCED_FACE('',(#6841),#759,.T.);
#25666=ADVANCED_FACE('',(#6842),#6506,.T.);
#25667=ADVANCED_FACE('',(#6843),#760,.T.);
#25668=ADVANCED_FACE('',(#6844,#619,#620),#761,.F.);
#25669=ADVANCED_FACE('',(#6845),#6507,.T.);
#25670=ADVANCED_FACE('',(#6846),#588,.F.);
#25671=ADVANCED_FACE('',(#6847),#6508,.T.);
#25672=ADVANCED_FACE('',(#6848),#589,.F.);
#25673=ADVANCED_FACE('',(#6849),#6509,.T.);
#25674=ADVANCED_FACE('',(#6850),#590,.F.);
#25675=ADVANCED_FACE('',(#6851),#6510,.T.);
#25676=ADVANCED_FACE('',(#6852),#591,.F.);
#25677=ADVANCED_FACE('',(#6853),#762,.T.);
#25678=ADVANCED_FACE('',(#6854),#6511,.T.);
#25679=ADVANCED_FACE('',(#6855),#763,.T.);
#25680=ADVANCED_FACE('',(#6856,#621,#622,#623),#764,.T.);
#25681=ADVANCED_FACE('',(#6857),#6512,.T.);
#25682=ADVANCED_FACE('',(#6858),#592,.F.);
#25683=ADVANCED_FACE('',(#6859),#6513,.T.);
#25684=ADVANCED_FACE('',(#6860),#593,.F.);
#25685=ADVANCED_FACE('',(#6861),#6514,.T.);
#25686=ADVANCED_FACE('',(#6862),#594,.F.);
#25687=ADVANCED_FACE('',(#6863),#6515,.T.);
#25688=ADVANCED_FACE('',(#6864),#595,.F.);
#25689=ADVANCED_FACE('',(#6865),#6516,.T.);
#25690=ADVANCED_FACE('',(#6866),#765,.T.);
#25691=ADVANCED_FACE('',(#6867),#6517,.T.);
#25692=ADVANCED_FACE('',(#6868),#766,.T.);
#25693=ADVANCED_FACE('',(#6869,#624),#767,.T.);
#25694=ADVANCED_FACE('',(#6870),#6518,.T.);
#25695=ADVANCED_FACE('',(#6871),#596,.F.);
#25696=ADVANCED_FACE('',(#6872),#6519,.T.);
#25697=ADVANCED_FACE('',(#6873),#597,.F.);
#25698=ADVANCED_FACE('',(#6874),#6520,.T.);
#25699=ADVANCED_FACE('',(#6875),#598,.F.);
#25700=ADVANCED_FACE('',(#6876),#6521,.T.);
#25701=ADVANCED_FACE('',(#6877),#599,.F.);
#25702=ADVANCED_FACE('',(#6878),#6522,.T.);
#25703=ADVANCED_FACE('',(#6879),#768,.T.);
#25704=ADVANCED_FACE('',(#6880),#6523,.T.);
#25705=ADVANCED_FACE('',(#6881),#769,.T.);
#25706=ADVANCED_FACE('',(#6882,#625),#770,.T.);
#25707=ADVANCED_FACE('',(#6883),#25598,.T.);
#25708=ADVANCED_FACE('',(#6884),#6524,.F.);
#25709=ADVANCED_FACE('',(#6885),#25599,.T.);
#25710=ADVANCED_FACE('',(#6886,#626),#771,.F.);
#25711=ADVANCED_FACE('',(#6887),#6525,.F.);
#25712=ADVANCED_FACE('',(#6888),#6526,.T.);
#25713=ADVANCED_FACE('',(#6889),#25600,.T.);
#25714=ADVANCED_FACE('',(#6890),#6527,.T.);
#25715=ADVANCED_FACE('',(#6891),#772,.F.);
#25716=ADVANCED_FACE('',(#6892),#6528,.T.);
#25717=ADVANCED_FACE('',(#6893),#773,.F.);
#25718=ADVANCED_FACE('',(#6894),#25601,.T.);
#25719=ADVANCED_FACE('',(#6895),#492,.F.);
#25720=ADVANCED_FACE('',(#6896),#25602,.T.);
#25721=ADVANCED_FACE('',(#6897),#493,.F.);
#25722=ADVANCED_FACE('',(#6898),#6529,.T.);
#25723=ADVANCED_FACE('',(#6899),#774,.T.);
#25724=ADVANCED_FACE('',(#6900),#6530,.F.);
#25725=ADVANCED_FACE('',(#6901),#6531,.T.);
#25726=ADVANCED_FACE('',(#6902),#6532,.T.);
#25727=ADVANCED_FACE('',(#6903),#25603,.T.);
#25728=ADVANCED_FACE('',(#6904),#6533,.T.);
#25729=ADVANCED_FACE('',(#6905),#25604,.T.);
#25730=ADVANCED_FACE('',(#6906),#6534,.T.);
#25731=ADVANCED_FACE('',(#6907),#775,.T.);
#25732=ADVANCED_FACE('',(#6908),#776,.F.);
#25733=ADVANCED_FACE('',(#6909),#6535,.T.);
#25734=ADVANCED_FACE('',(#6910),#25605,.T.);
#25735=ADVANCED_FACE('',(#6911),#6536,.T.);
#25736=ADVANCED_FACE('',(#6912),#25606,.T.);
#25737=ADVANCED_FACE('',(#6913),#6537,.T.);
#25738=ADVANCED_FACE('',(#6914),#25607,.T.);
#25739=ADVANCED_FACE('',(#6915),#6538,.T.);
#25740=ADVANCED_FACE('',(#6916),#25608,.T.);
#25741=ADVANCED_FACE('',(#6917),#777,.T.);
#25742=ADVANCED_FACE('',(#6918,#627,#628,#629),#778,.T.);
#25743=ADVANCED_FACE('',(#6919),#25609,.T.);
#25744=ADVANCED_FACE('',(#6920),#494,.F.);
#25745=ADVANCED_FACE('',(#6921),#25610,.T.);
#25746=ADVANCED_FACE('',(#6922),#495,.F.);
#25747=ADVANCED_FACE('',(#6923),#6539,.T.);
#25748=ADVANCED_FACE('',(#6924),#6540,.F.);
#25749=ADVANCED_FACE('',(#6925),#6541,.F.);
#25750=ADVANCED_FACE('',(#6926),#6542,.F.);
#25751=ADVANCED_FACE('',(#6927),#6543,.F.);
#25752=ADVANCED_FACE('',(#6928),#779,.T.);
#25753=ADVANCED_FACE('',(#6929),#6544,.F.);
#25754=ADVANCED_FACE('',(#6930),#780,.T.);
#25755=ADVANCED_FACE('',(#6931),#6545,.F.);
#25756=ADVANCED_FACE('',(#6932),#781,.T.);
#25757=ADVANCED_FACE('',(#6933),#782,.F.);
#25758=ADVANCED_FACE('',(#6934),#783,.T.);
#25759=ADVANCED_FACE('',(#6935),#784,.T.);
#25760=ADVANCED_FACE('',(#6936),#785,.T.);
#25761=ADVANCED_FACE('',(#6937),#6546,.F.);
#25762=ADVANCED_FACE('',(#6938),#786,.T.);
#25763=ADVANCED_FACE('',(#6939),#6547,.F.);
#25764=ADVANCED_FACE('',(#6940),#787,.T.);
#25765=ADVANCED_FACE('',(#6941),#6548,.F.);
#25766=ADVANCED_FACE('',(#6942),#788,.T.);
#25767=ADVANCED_FACE('',(#6943),#6549,.F.);
#25768=ADVANCED_FACE('',(#6944),#789,.T.);
#25769=ADVANCED_FACE('',(#6945),#6550,.F.);
#25770=ADVANCED_FACE('',(#6946),#790,.F.);
#25771=ADVANCED_FACE('',(#6947),#6551,.F.);
#25772=ADVANCED_FACE('',(#6948),#791,.F.);
#25773=ADVANCED_FACE('',(#6949),#6552,.F.);
#25774=ADVANCED_FACE('',(#6950),#792,.F.);
#25775=ADVANCED_FACE('',(#6951),#6553,.F.);
#25776=ADVANCED_FACE('',(#6952),#793,.F.);
#25777=ADVANCED_FACE('',(#6953),#6554,.F.);
#25778=ADVANCED_FACE('',(#6954),#794,.F.);
#25779=ADVANCED_FACE('',(#6955),#6555,.F.);
#25780=ADVANCED_FACE('',(#6956),#795,.F.);
#25781=ADVANCED_FACE('',(#6957),#6556,.F.);
#25782=ADVANCED_FACE('',(#6958),#796,.F.);
#25783=ADVANCED_FACE('',(#6959),#6557,.F.);
#25784=ADVANCED_FACE('',(#6960),#797,.F.);
#25785=ADVANCED_FACE('',(#6961),#798,.F.);
#25786=ADVANCED_FACE('',(#6962,#630),#799,.F.);
#25787=ADVANCED_FACE('',(#6963),#6558,.F.);
#25788=ADVANCED_FACE('',(#6964),#6559,.T.);
#25789=ADVANCED_FACE('',(#6965),#800,.T.);
#25790=ADVANCED_FACE('',(#6966),#6560,.T.);
#25791=ADVANCED_FACE('',(#6967),#801,.T.);
#25792=ADVANCED_FACE('',(#6968),#6561,.T.);
#25793=ADVANCED_FACE('',(#6969),#802,.T.);
#25794=ADVANCED_FACE('',(#6970),#6562,.T.);
#25795=ADVANCED_FACE('',(#6971),#803,.T.);
#25796=ADVANCED_FACE('',(#6972),#6563,.T.);
#25797=ADVANCED_FACE('',(#6973),#6564,.T.);
#25798=ADVANCED_FACE('',(#6974),#804,.T.);
#25799=ADVANCED_FACE('',(#6975),#6565,.T.);
#25800=ADVANCED_FACE('',(#6976),#805,.T.);
#25801=ADVANCED_FACE('',(#6977),#6566,.T.);
#25802=ADVANCED_FACE('',(#6978),#806,.T.);
#25803=ADVANCED_FACE('',(#6979),#6567,.T.);
#25804=ADVANCED_FACE('',(#6980),#807,.T.);
#25805=ADVANCED_FACE('',(#6981),#808,.F.);
#25806=ADVANCED_FACE('',(#6982),#809,.T.);
#25807=ADVANCED_FACE('',(#6983),#6568,.T.);
#27221=CLOSED_SHELL('',(#25651,#25652,#25653,#25654,#25655,#25656,#25657,
#25658,#25659,#25660,#25661,#25662,#25663,#25664,#25665,#25666,#25667,#25668,
#25669,#25670,#25671,#25672,#25673,#25674,#25675,#25676,#25677,#25678,#25679,
#25680,#25681,#25682,#25683,#25684,#25685,#25686,#25687,#25688,#25689,#25690,
#25691,#25692,#25693,#25694,#25695,#25696,#25697,#25698,#25699,#25700,#25701,
#25702,#25703,#25704,#25705,#25706,#25707,#25708,#25709,#25710,#25711,#25712,
#25713,#25714,#25715,#25716,#25717,#25718,#25719,#25720,#25721,#25722,#25723,
#25724,#25725,#25726,#25727,#25728,#25729,#25730,#25731,#25732,#25733,#25734,
#25735,#25736,#25737,#25738,#25739,#25740,#25741,#25742,#25743,#25744,#25745,
#25746,#25747,#25748,#25749,#25750,#25751,#25752,#25753,#25754,#25755,#25756,
#25757,#25758,#25759,#25760,#25761,#25762,#25763,#25764,#25765,#25766,#25767,
#25768,#25769,#25770,#25771,#25772,#25773,#25774,#25775,#25776,#25777,#25778,
#25779,#25780,#25781,#25782,#25783,#25784,#25785,#25786,#25787,#25788,#25789,
#25790,#25791,#25792,#25793,#25794,#25795,#25796,#25797,#25798,#25799,#25800,
#25801,#25802,#25803,#25804,#25805,#25806,#25807));
#27463=AXIS2_PLACEMENT_3D('',#37376,#29978,#29979);
#27464=AXIS2_PLACEMENT_3D('',#37377,#29980,#29981);
#27465=AXIS2_PLACEMENT_3D('',#37387,#29982,#29983);
#27466=AXIS2_PLACEMENT_3D('',#37389,#29984,#29985);
#27467=AXIS2_PLACEMENT_3D('',#37390,#29986,#29987);
#27468=AXIS2_PLACEMENT_3D('',#37392,#29988,#29989);
#27469=AXIS2_PLACEMENT_3D('',#37412,#29990,#29991);
#27470=AXIS2_PLACEMENT_3D('',#37413,#29992,#29993);
#27471=AXIS2_PLACEMENT_3D('',#37417,#29995,#29996);
#27472=AXIS2_PLACEMENT_3D('',#37419,#29997,#29998);
#27473=AXIS2_PLACEMENT_3D('',#37445,#30000,#30001);
#27474=AXIS2_PLACEMENT_3D('',#37471,#30003,#30004);
#27475=AXIS2_PLACEMENT_3D('',#37491,#30006,#30007);
#27476=AXIS2_PLACEMENT_3D('',#37493,#30008,#30009);
#27477=AXIS2_PLACEMENT_3D('',#37495,#30010,#30011);
#27478=AXIS2_PLACEMENT_3D('',#37497,#30012,#30013);
#27479=AXIS2_PLACEMENT_3D('',#37499,#30014,#30015);
#27480=AXIS2_PLACEMENT_3D('',#37501,#30016,#30017);
#27481=AXIS2_PLACEMENT_3D('',#37502,#30018,#30019);
#27482=AXIS2_PLACEMENT_3D('',#37504,#30020,#30021);
#27483=AXIS2_PLACEMENT_3D('',#37505,#30022,#30023);
#27484=AXIS2_PLACEMENT_3D('',#37506,#30024,#30025);
#27485=AXIS2_PLACEMENT_3D('',#37507,#30026,#30027);
#27486=AXIS2_PLACEMENT_3D('',#37508,#30028,#30029);
#27487=AXIS2_PLACEMENT_3D('',#37510,#30030,#30031);
#27488=AXIS2_PLACEMENT_3D('',#37512,#30032,#30033);
#27489=AXIS2_PLACEMENT_3D('',#37514,#30034,#30035);
#27490=AXIS2_PLACEMENT_3D('',#37516,#30036,#30037);
#27491=AXIS2_PLACEMENT_3D('',#37518,#30038,#30039);
#27492=AXIS2_PLACEMENT_3D('',#37520,#30040,#30041);
#27493=AXIS2_PLACEMENT_3D('',#37522,#30042,#30043);
#27494=AXIS2_PLACEMENT_3D('',#37524,#30044,#30045);
#27495=AXIS2_PLACEMENT_3D('',#37526,#30046,#30047);
#27496=AXIS2_PLACEMENT_3D('',#37527,#30048,#30049);
#27497=AXIS2_PLACEMENT_3D('',#37530,#30050,#30051);
#27498=AXIS2_PLACEMENT_3D('',#37534,#30053,#30054);
#27499=AXIS2_PLACEMENT_3D('',#37547,#30056,#30057);
#27500=AXIS2_PLACEMENT_3D('',#37548,#30058,#30059);
#27501=AXIS2_PLACEMENT_3D('',#37549,#30060,#30061);
#27502=AXIS2_PLACEMENT_3D('',#37550,#30062,#30063);
#27503=AXIS2_PLACEMENT_3D('',#37553,#30064,#30065);
#27504=AXIS2_PLACEMENT_3D('',#37567,#30068,#30069);
#27505=AXIS2_PLACEMENT_3D('',#37568,#30070,#30071);
#27506=AXIS2_PLACEMENT_3D('',#37569,#30072,#30073);
#27507=AXIS2_PLACEMENT_3D('',#37570,#30074,#30075);
#27508=AXIS2_PLACEMENT_3D('',#37573,#30076,#30077);
#27509=AXIS2_PLACEMENT_3D('',#37587,#30080,#30081);
#27510=AXIS2_PLACEMENT_3D('',#37588,#30082,#30083);
#27511=AXIS2_PLACEMENT_3D('',#37589,#30084,#30085);
#27512=AXIS2_PLACEMENT_3D('',#37590,#30086,#30087);
#27513=AXIS2_PLACEMENT_3D('',#37593,#30088,#30089);
#27514=AXIS2_PLACEMENT_3D('',#37605,#30092,#30093);
#27515=AXIS2_PLACEMENT_3D('',#37606,#30094,#30095);
#27516=AXIS2_PLACEMENT_3D('',#37607,#30096,#30097);
#27517=AXIS2_PLACEMENT_3D('',#37611,#30099,#30100);
#27518=AXIS2_PLACEMENT_3D('',#37613,#30102,#30103);
#27519=AXIS2_PLACEMENT_3D('',#37617,#30106,#30107);
#27520=AXIS2_PLACEMENT_3D('',#37620,#30109,#30110);
#27521=AXIS2_PLACEMENT_3D('',#37621,#30111,#30112);
#27522=AXIS2_PLACEMENT_3D('',#37625,#30115,#30116);
#27523=AXIS2_PLACEMENT_3D('',#37627,#30117,#30118);
#27524=AXIS2_PLACEMENT_3D('',#37629,#30119,#30120);
#27525=AXIS2_PLACEMENT_3D('',#37630,#30121,#30122);
#27526=AXIS2_PLACEMENT_3D('',#37633,#30123,#30124);
#27527=AXIS2_PLACEMENT_3D('',#37637,#30126,#30127);
#27528=AXIS2_PLACEMENT_3D('',#37650,#30129,#30130);
#27529=AXIS2_PLACEMENT_3D('',#37651,#30131,#30132);
#27530=AXIS2_PLACEMENT_3D('',#37652,#30133,#30134);
#27531=AXIS2_PLACEMENT_3D('',#37653,#30135,#30136);
#27532=AXIS2_PLACEMENT_3D('',#37655,#30137,#30138);
#27533=AXIS2_PLACEMENT_3D('',#37668,#30141,#30142);
#27534=AXIS2_PLACEMENT_3D('',#37669,#30143,#30144);
#27535=AXIS2_PLACEMENT_3D('',#37670,#30145,#30146);
#27536=AXIS2_PLACEMENT_3D('',#37672,#30147,#30148);
#27537=AXIS2_PLACEMENT_3D('',#37684,#30150,#30151);
#27538=AXIS2_PLACEMENT_3D('',#37685,#30152,#30153);
#27539=AXIS2_PLACEMENT_3D('',#37686,#30154,#30155);
#27540=AXIS2_PLACEMENT_3D('',#37688,#30156,#30157);
#27541=AXIS2_PLACEMENT_3D('',#37699,#30159,#30160);
#27542=AXIS2_PLACEMENT_3D('',#37700,#30161,#30162);
#27543=AXIS2_PLACEMENT_3D('',#37701,#30163,#30164);
#27544=AXIS2_PLACEMENT_3D('',#37703,#30166,#30167);
#27545=AXIS2_PLACEMENT_3D('',#37705,#30169,#30170);
#27546=AXIS2_PLACEMENT_3D('',#37707,#30172,#30173);
#27547=AXIS2_PLACEMENT_3D('',#37710,#30174,#30175);
#27548=AXIS2_PLACEMENT_3D('',#37714,#30177,#30178);
#27549=AXIS2_PLACEMENT_3D('',#37718,#30180,#30181);
#27550=AXIS2_PLACEMENT_3D('',#37722,#30183,#30184);
#27551=AXIS2_PLACEMENT_3D('',#37725,#30186,#30187);
#27552=AXIS2_PLACEMENT_3D('',#37727,#30188,#30189);
#27553=AXIS2_PLACEMENT_3D('',#37728,#30190,#30191);
#27554=AXIS2_PLACEMENT_3D('',#37731,#30192,#30193);
#27555=AXIS2_PLACEMENT_3D('',#37735,#30195,#30196);
#27556=AXIS2_PLACEMENT_3D('',#37748,#30198,#30199);
#27557=AXIS2_PLACEMENT_3D('',#37749,#30200,#30201);
#27558=AXIS2_PLACEMENT_3D('',#37750,#30202,#30203);
#27559=AXIS2_PLACEMENT_3D('',#37751,#30204,#30205);
#27560=AXIS2_PLACEMENT_3D('',#37754,#30206,#30207);
#27561=AXIS2_PLACEMENT_3D('',#37768,#30210,#30211);
#27562=AXIS2_PLACEMENT_3D('',#37769,#30212,#30213);
#27563=AXIS2_PLACEMENT_3D('',#37770,#30214,#30215);
#27564=AXIS2_PLACEMENT_3D('',#37771,#30216,#30217);
#27565=AXIS2_PLACEMENT_3D('',#37774,#30218,#30219);
#27566=AXIS2_PLACEMENT_3D('',#37788,#30222,#30223);
#27567=AXIS2_PLACEMENT_3D('',#37789,#30224,#30225);
#27568=AXIS2_PLACEMENT_3D('',#37790,#30226,#30227);
#27569=AXIS2_PLACEMENT_3D('',#37791,#30228,#30229);
#27570=AXIS2_PLACEMENT_3D('',#37794,#30230,#30231);
#27571=AXIS2_PLACEMENT_3D('',#37806,#30234,#30235);
#27572=AXIS2_PLACEMENT_3D('',#37807,#30236,#30237);
#27573=AXIS2_PLACEMENT_3D('',#37808,#30238,#30239);
#27574=AXIS2_PLACEMENT_3D('',#37812,#30241,#30242);
#27575=AXIS2_PLACEMENT_3D('',#37814,#30244,#30245);
#27576=AXIS2_PLACEMENT_3D('',#37818,#30248,#30249);
#27577=AXIS2_PLACEMENT_3D('',#37821,#30251,#30252);
#27578=AXIS2_PLACEMENT_3D('',#37822,#30253,#30254);
#27579=AXIS2_PLACEMENT_3D('',#37826,#30257,#30258);
#27580=AXIS2_PLACEMENT_3D('',#37828,#30259,#30260);
#27581=AXIS2_PLACEMENT_3D('',#37829,#30261,#30262);
#27582=AXIS2_PLACEMENT_3D('',#37832,#30263,#30264);
#27583=AXIS2_PLACEMENT_3D('',#37836,#30266,#30267);
#27584=AXIS2_PLACEMENT_3D('',#37849,#30269,#30270);
#27585=AXIS2_PLACEMENT_3D('',#37850,#30271,#30272);
#27586=AXIS2_PLACEMENT_3D('',#37851,#30273,#30274);
#27587=AXIS2_PLACEMENT_3D('',#37852,#30275,#30276);
#27588=AXIS2_PLACEMENT_3D('',#37855,#30277,#30278);
#27589=AXIS2_PLACEMENT_3D('',#37869,#30281,#30282);
#27590=AXIS2_PLACEMENT_3D('',#37870,#30283,#30284);
#27591=AXIS2_PLACEMENT_3D('',#37871,#30285,#30286);
#27592=AXIS2_PLACEMENT_3D('',#37872,#30287,#30288);
#27593=AXIS2_PLACEMENT_3D('',#37875,#30289,#30290);
#27594=AXIS2_PLACEMENT_3D('',#37889,#30293,#30294);
#27595=AXIS2_PLACEMENT_3D('',#37890,#30295,#30296);
#27596=AXIS2_PLACEMENT_3D('',#37891,#30297,#30298);
#27597=AXIS2_PLACEMENT_3D('',#37892,#30299,#30300);
#27598=AXIS2_PLACEMENT_3D('',#37895,#30301,#30302);
#27599=AXIS2_PLACEMENT_3D('',#37907,#30305,#30306);
#27600=AXIS2_PLACEMENT_3D('',#37908,#30307,#30308);
#27601=AXIS2_PLACEMENT_3D('',#37909,#30309,#30310);
#27602=AXIS2_PLACEMENT_3D('',#37913,#30312,#30313);
#27603=AXIS2_PLACEMENT_3D('',#37915,#30315,#30316);
#27604=AXIS2_PLACEMENT_3D('',#37919,#30319,#30320);
#27605=AXIS2_PLACEMENT_3D('',#37922,#30322,#30323);
#27606=AXIS2_PLACEMENT_3D('',#37923,#30324,#30325);
#27607=AXIS2_PLACEMENT_3D('',#37927,#30328,#30329);
#27608=AXIS2_PLACEMENT_3D('',#37929,#30330,#30331);
#27609=AXIS2_PLACEMENT_3D('',#37930,#30332,#30333);
#27610=AXIS2_PLACEMENT_3D('',#37932,#30334,#30335);
#27611=AXIS2_PLACEMENT_3D('',#37933,#30336,#30337);
#27612=AXIS2_PLACEMENT_3D('',#37934,#30338,#30339);
#27613=AXIS2_PLACEMENT_3D('',#37938,#30341,#30342);
#27614=AXIS2_PLACEMENT_3D('',#37953,#30344,#30345);
#27615=AXIS2_PLACEMENT_3D('',#37967,#30347,#30348);
#27616=AXIS2_PLACEMENT_3D('',#37968,#30349,#30350);
#27617=AXIS2_PLACEMENT_3D('',#37970,#30351,#30352);
#27618=AXIS2_PLACEMENT_3D('',#37972,#30353,#30354);
#27619=AXIS2_PLACEMENT_3D('',#37973,#30355,#30356);
#27620=AXIS2_PLACEMENT_3D('',#37974,#30357,#30358);
#27621=AXIS2_PLACEMENT_3D('',#37979,#30361,#30362);
#27622=AXIS2_PLACEMENT_3D('',#37980,#30363,#30364);
#27623=AXIS2_PLACEMENT_3D('',#37983,#30366,#30367);
#27624=AXIS2_PLACEMENT_3D('',#37984,#30368,#30369);
#27625=AXIS2_PLACEMENT_3D('',#38001,#30371,#30372);
#27626=AXIS2_PLACEMENT_3D('',#38003,#30373,#30374);
#27627=AXIS2_PLACEMENT_3D('',#38018,#30375,#30376);
#27628=AXIS2_PLACEMENT_3D('',#38020,#30378,#30379);
#27629=AXIS2_PLACEMENT_3D('',#38024,#30382,#30383);
#27630=AXIS2_PLACEMENT_3D('',#38027,#30385,#30386);
#27631=AXIS2_PLACEMENT_3D('',#38028,#30387,#30388);
#27632=AXIS2_PLACEMENT_3D('',#38030,#30390,#30391);
#27633=AXIS2_PLACEMENT_3D('',#38033,#30392,#30393);
#27634=AXIS2_PLACEMENT_3D('',#38035,#30394,#30395);
#27635=AXIS2_PLACEMENT_3D('',#38037,#30396,#30397);
#27636=AXIS2_PLACEMENT_3D('',#38039,#30398,#30399);
#27637=AXIS2_PLACEMENT_3D('',#38040,#30400,#30401);
#27638=AXIS2_PLACEMENT_3D('',#38091,#30402,#30403);
#27639=AXIS2_PLACEMENT_3D('',#38108,#30404,#30405);
#27640=AXIS2_PLACEMENT_3D('',#38111,#30406,#30407);
#27641=AXIS2_PLACEMENT_3D('',#38112,#30408,#30409);
#27642=AXIS2_PLACEMENT_3D('',#38113,#30410,#30411);
#27643=AXIS2_PLACEMENT_3D('',#38178,#30412,#30413);
#27644=AXIS2_PLACEMENT_3D('',#38182,#30415,#30416);
#27645=AXIS2_PLACEMENT_3D('',#38186,#30418,#30419);
#27646=AXIS2_PLACEMENT_3D('',#38188,#30421,#30422);
#27647=AXIS2_PLACEMENT_3D('',#38192,#30425,#30426);
#27648=AXIS2_PLACEMENT_3D('',#38195,#30428,#30429);
#27649=AXIS2_PLACEMENT_3D('',#38196,#30430,#30431);
#27650=AXIS2_PLACEMENT_3D('',#38200,#30433,#30434);
#27651=AXIS2_PLACEMENT_3D('',#38202,#30436,#30437);
#27652=AXIS2_PLACEMENT_3D('',#38205,#30438,#30439);
#27653=AXIS2_PLACEMENT_3D('',#38209,#30441,#30442);
#27654=AXIS2_PLACEMENT_3D('',#38211,#30444,#30445);
#27655=AXIS2_PLACEMENT_3D('',#38214,#30446,#30447);
#27656=AXIS2_PLACEMENT_3D('',#38215,#30448,#30449);
#27657=AXIS2_PLACEMENT_3D('',#38216,#30450,#30451);
#27658=AXIS2_PLACEMENT_3D('',#38217,#30452,#30453);
#27659=AXIS2_PLACEMENT_3D('',#38220,#30456,#30457);
#27660=AXIS2_PLACEMENT_3D('',#38221,#30458,#30459);
#27661=AXIS2_PLACEMENT_3D('',#38222,#30460,#30461);
#27662=AXIS2_PLACEMENT_3D('',#38223,#30462,#30463);
#27663=AXIS2_PLACEMENT_3D('',#38227,#30465,#30466);
#27664=AXIS2_PLACEMENT_3D('',#38241,#30469,#30470);
#27665=AXIS2_PLACEMENT_3D('',#38244,#30473,#30474);
#27666=AXIS2_PLACEMENT_3D('',#38245,#30475,#30476);
#27667=AXIS2_PLACEMENT_3D('',#38248,#30477,#30478);
#27668=AXIS2_PLACEMENT_3D('',#38251,#30480,#30481);
#27669=AXIS2_PLACEMENT_3D('',#38253,#30483,#30484);
#27670=AXIS2_PLACEMENT_3D('',#38255,#30485,#30486);
#27671=AXIS2_PLACEMENT_3D('',#38256,#30487,#30488);
#27672=AXIS2_PLACEMENT_3D('',#38257,#30489,#30490);
#27673=AXIS2_PLACEMENT_3D('',#38259,#30491,#30492);
#27674=AXIS2_PLACEMENT_3D('',#38261,#30494,#30495);
#27675=AXIS2_PLACEMENT_3D('',#38263,#30496,#30497);
#27676=AXIS2_PLACEMENT_3D('',#38264,#30498,#30499);
#27677=AXIS2_PLACEMENT_3D('',#38265,#30500,#30501);
#27678=AXIS2_PLACEMENT_3D('',#38267,#30502,#30503);
#27679=AXIS2_PLACEMENT_3D('',#38269,#30505,#30506);
#27680=AXIS2_PLACEMENT_3D('',#38272,#30507,#30508);
#27681=AXIS2_PLACEMENT_3D('',#38273,#30509,#30510);
#27682=AXIS2_PLACEMENT_3D('',#38274,#30511,#30512);
#27683=AXIS2_PLACEMENT_3D('',#38275,#30513,#30514);
#27684=AXIS2_PLACEMENT_3D('',#38278,#30515,#30516);
#27685=AXIS2_PLACEMENT_3D('',#38281,#30519,#30520);
#27686=AXIS2_PLACEMENT_3D('',#38282,#30521,#30522);
#27687=AXIS2_PLACEMENT_3D('',#38283,#30523,#30524);
#27688=AXIS2_PLACEMENT_3D('',#38284,#30525,#30526);
#27689=AXIS2_PLACEMENT_3D('',#38287,#30528,#30529);
#27690=AXIS2_PLACEMENT_3D('',#38288,#30530,#30531);
#27691=AXIS2_PLACEMENT_3D('',#38290,#30532,#30533);
#27692=AXIS2_PLACEMENT_3D('',#38294,#30535,#30536);
#27693=AXIS2_PLACEMENT_3D('',#38297,#30538,#30539);
#27694=AXIS2_PLACEMENT_3D('',#38301,#30541,#30542);
#27695=AXIS2_PLACEMENT_3D('',#38304,#30544,#30545);
#27696=AXIS2_PLACEMENT_3D('',#38305,#30546,#30547);
#27697=AXIS2_PLACEMENT_3D('',#38307,#30548,#30549);
#27698=AXIS2_PLACEMENT_3D('',#38309,#30550,#30551);
#27699=AXIS2_PLACEMENT_3D('',#38311,#30552,#30553);
#27700=AXIS2_PLACEMENT_3D('',#38312,#30554,#30555);
#27701=AXIS2_PLACEMENT_3D('',#38368,#30556,#30557);
#27702=AXIS2_PLACEMENT_3D('',#38378,#30558,#30559);
#27703=AXIS2_PLACEMENT_3D('',#38381,#30560,#30561);
#27704=AXIS2_PLACEMENT_3D('',#38382,#30562,#30563);
#27705=AXIS2_PLACEMENT_3D('',#38383,#30564,#30565);
#27706=AXIS2_PLACEMENT_3D('',#38448,#30566,#30567);
#27707=AXIS2_PLACEMENT_3D('',#38451,#30570,#30571);
#27708=AXIS2_PLACEMENT_3D('',#38454,#30573,#30574);
#27709=AXIS2_PLACEMENT_3D('',#38455,#30575,#30576);
#27710=AXIS2_PLACEMENT_3D('',#38457,#30578,#30579);
#27711=AXIS2_PLACEMENT_3D('',#38459,#30581,#30582);
#27712=AXIS2_PLACEMENT_3D('',#38462,#30584,#30585);
#27713=AXIS2_PLACEMENT_3D('',#38463,#30586,#30587);
#27714=AXIS2_PLACEMENT_3D('',#38464,#30588,#30589);
#27715=AXIS2_PLACEMENT_3D('',#38467,#30591,#30592);
#27716=AXIS2_PLACEMENT_3D('',#38468,#30593,#30594);
#27717=AXIS2_PLACEMENT_3D('',#38469,#30595,#30596);
#27718=AXIS2_PLACEMENT_3D('',#38472,#30598,#30599);
#27719=AXIS2_PLACEMENT_3D('',#38473,#30600,#30601);
#27720=AXIS2_PLACEMENT_3D('',#38474,#30602,#30603);
#27721=AXIS2_PLACEMENT_3D('',#38475,#30604,#30605);
#27722=AXIS2_PLACEMENT_3D('',#38476,#30606,#30607);
#27723=AXIS2_PLACEMENT_3D('',#38477,#30608,#30609);
#27724=AXIS2_PLACEMENT_3D('',#38481,#30612,#30613);
#27725=AXIS2_PLACEMENT_3D('',#38484,#30615,#30616);
#27726=AXIS2_PLACEMENT_3D('',#38485,#30617,#30618);
#27727=AXIS2_PLACEMENT_3D('',#38486,#30619,#30620);
#27728=AXIS2_PLACEMENT_3D('',#38489,#30622,#30623);
#27729=AXIS2_PLACEMENT_3D('',#38490,#30624,#30625);
#27730=AXIS2_PLACEMENT_3D('',#38491,#30626,#30627);
#27731=AXIS2_PLACEMENT_3D('',#38494,#30629,#30630);
#27732=AXIS2_PLACEMENT_3D('',#38495,#30631,#30632);
#27733=AXIS2_PLACEMENT_3D('',#38496,#30633,#30634);
#27734=AXIS2_PLACEMENT_3D('',#38499,#30636,#30637);
#27735=AXIS2_PLACEMENT_3D('',#38500,#30638,#30639);
#27736=AXIS2_PLACEMENT_3D('',#38501,#30640,#30641);
#27737=AXIS2_PLACEMENT_3D('',#38504,#30643,#30644);
#27738=AXIS2_PLACEMENT_3D('',#38505,#30645,#30646);
#27739=AXIS2_PLACEMENT_3D('',#38506,#30647,#30648);
#27740=AXIS2_PLACEMENT_3D('',#38509,#30650,#30651);
#27741=AXIS2_PLACEMENT_3D('',#38510,#30652,#30653);
#27742=AXIS2_PLACEMENT_3D('',#38511,#30654,#30655);
#27743=AXIS2_PLACEMENT_3D('',#38514,#30657,#30658);
#27744=AXIS2_PLACEMENT_3D('',#38515,#30659,#30660);
#27745=AXIS2_PLACEMENT_3D('',#38516,#30661,#30662);
#27746=AXIS2_PLACEMENT_3D('',#38519,#30664,#30665);
#27747=AXIS2_PLACEMENT_3D('',#38520,#30666,#30667);
#27748=AXIS2_PLACEMENT_3D('',#38521,#30668,#30669);
#27749=AXIS2_PLACEMENT_3D('',#38524,#30671,#30672);
#27750=AXIS2_PLACEMENT_3D('',#38525,#30673,#30674);
#27751=AXIS2_PLACEMENT_3D('',#38526,#30675,#30676);
#27752=AXIS2_PLACEMENT_3D('',#38529,#30678,#30679);
#27753=AXIS2_PLACEMENT_3D('',#38530,#30680,#30681);
#27754=AXIS2_PLACEMENT_3D('',#38531,#30682,#30683);
#27755=AXIS2_PLACEMENT_3D('',#38534,#30685,#30686);
#27756=AXIS2_PLACEMENT_3D('',#38535,#30687,#30688);
#27757=AXIS2_PLACEMENT_3D('',#38536,#30689,#30690);
#27758=AXIS2_PLACEMENT_3D('',#38539,#30692,#30693);
#27759=AXIS2_PLACEMENT_3D('',#38540,#30694,#30695);
#27760=AXIS2_PLACEMENT_3D('',#38541,#30696,#30697);
#27761=AXIS2_PLACEMENT_3D('',#38542,#30698,#30699);
#27762=AXIS2_PLACEMENT_3D('',#38544,#30700,#30701);
#27763=AXIS2_PLACEMENT_3D('',#38545,#30702,#30703);
#27764=AXIS2_PLACEMENT_3D('',#38547,#30705,#30706);
#27765=AXIS2_PLACEMENT_3D('',#38549,#30708,#30709);
#27766=AXIS2_PLACEMENT_3D('',#38551,#30711,#30712);
#27767=AXIS2_PLACEMENT_3D('',#38553,#30714,#30715);
#27768=AXIS2_PLACEMENT_3D('',#38554,#30716,#30717);
#27769=AXIS2_PLACEMENT_3D('',#38556,#30719,#30720);
#27770=AXIS2_PLACEMENT_3D('',#38558,#30722,#30723);
#27771=AXIS2_PLACEMENT_3D('',#38560,#30725,#30726);
#27772=AXIS2_PLACEMENT_3D('',#38561,#30727,#30728);
#27773=AXIS2_PLACEMENT_3D('',#38562,#30729,#30730);
#27774=AXIS2_PLACEMENT_3D('',#38565,#30733,#30734);
#27775=AXIS2_PLACEMENT_3D('',#38567,#30736,#30737);
#27776=AXIS2_PLACEMENT_3D('',#38569,#30739,#30740);
#27777=AXIS2_PLACEMENT_3D('',#38571,#30742,#30743);
#27778=AXIS2_PLACEMENT_3D('',#38573,#30745,#30746);
#27779=AXIS2_PLACEMENT_3D('',#38575,#30748,#30749);
#27780=AXIS2_PLACEMENT_3D('',#38577,#30751,#30752);
#27781=AXIS2_PLACEMENT_3D('',#38578,#30753,#30754);
#27782=AXIS2_PLACEMENT_3D('',#38581,#30756,#30757);
#27783=AXIS2_PLACEMENT_3D('',#38582,#30758,#30759);
#27784=AXIS2_PLACEMENT_3D('',#38584,#30761,#30762);
#29978=DIRECTION('axis',(0.,0.,1.));
#29979=DIRECTION('refdir',(1.,0.,0.));
#29980=DIRECTION('center_axis',(0.,-1.,0.));
#29981=DIRECTION('ref_axis',(0.,0.,1.));
#29982=DIRECTION('center_axis',(0.,1.,0.));
#29983=DIRECTION('ref_axis',(0.,0.,1.));
#29984=DIRECTION('center_axis',(1.,0.,-1.22464679914735E-16));
#29985=DIRECTION('ref_axis',(-1.22464679914735E-16,0.,-1.));
#29986=DIRECTION('center_axis',(0.,-1.,0.));
#29987=DIRECTION('ref_axis',(0.,0.,1.));
#29988=DIRECTION('center_axis',(0.,1.,0.));
#29989=DIRECTION('ref_axis',(0.,0.,1.));
#29990=DIRECTION('center_axis',(0.,-1.,0.));
#29991=DIRECTION('ref_axis',(0.,0.,-1.));
#29992=DIRECTION('center_axis',(0.,1.,0.));
#29993=DIRECTION('ref_axis',(-0.013060400300148,0.,-0.999914709334751));
#29994=DIRECTION('',(0.,-1.,0.));
#29995=DIRECTION('center_axis',(0.,-1.,0.));
#29996=DIRECTION('ref_axis',(-0.468970569827389,0.,0.883213793277581));
#29997=DIRECTION('center_axis',(0.,-1.,0.));
#29998=DIRECTION('ref_axis',(-0.468970569827389,0.,0.883213793277581));
#29999=DIRECTION('',(0.,1.,0.));
#30000=DIRECTION('center_axis',(0.,1.,0.));
#30001=DIRECTION('ref_axis',(0.,0.,1.));
#30002=DIRECTION('',(0.,-1.,0.));
#30003=DIRECTION('center_axis',(0.,-1.,0.));
#30004=DIRECTION('ref_axis',(-0.468970569827389,0.,0.883213793277581));
#30005=DIRECTION('',(0.,1.,0.));
#30006=DIRECTION('center_axis',(0.,1.,0.));
#30007=DIRECTION('ref_axis',(0.,0.,1.));
#30008=DIRECTION('center_axis',(0.,-1.,0.));
#30009=DIRECTION('ref_axis',(1.,0.,0.));
#30010=DIRECTION('center_axis',(0.,-1.,0.));
#30011=DIRECTION('ref_axis',(1.,0.,0.));
#30012=DIRECTION('center_axis',(0.,-1.,0.));
#30013=DIRECTION('ref_axis',(1.,0.,0.));
#30014=DIRECTION('center_axis',(0.,-1.,0.));
#30015=DIRECTION('ref_axis',(1.,0.,0.));
#30016=DIRECTION('center_axis',(0.,-1.,0.));
#30017=DIRECTION('ref_axis',(0.,0.,1.));
#30018=DIRECTION('center_axis',(0.,1.,0.));
#30019=DIRECTION('ref_axis',(-0.468970569827389,0.,0.883213793277581));
#30020=DIRECTION('center_axis',(-0.883213793277581,0.,-0.468970569827389));
#30021=DIRECTION('ref_axis',(0.468970569827389,0.,-0.883213793277581));
#30022=DIRECTION('center_axis',(0.,1.,0.));
#30023=DIRECTION('ref_axis',(-0.468970569827389,0.,0.883213793277581));
#30024=DIRECTION('center_axis',(0.,-1.,0.));
#30025=DIRECTION('ref_axis',(0.,0.,1.));
#30026=DIRECTION('center_axis',(0.,-1.,0.));
#30027=DIRECTION('ref_axis',(0.,0.,1.));
#30028=DIRECTION('center_axis',(0.,-1.,0.));
#30029=DIRECTION('ref_axis',(0.,0.,-1.));
#30030=DIRECTION('center_axis',(0.,1.,0.));
#30031=DIRECTION('ref_axis',(1.,0.,0.));
#30032=DIRECTION('center_axis',(0.,1.,0.));
#30033=DIRECTION('ref_axis',(1.,0.,0.));
#30034=DIRECTION('center_axis',(0.,1.,0.));
#30035=DIRECTION('ref_axis',(1.,0.,0.));
#30036=DIRECTION('center_axis',(0.,1.,0.));
#30037=DIRECTION('ref_axis',(1.,0.,0.));
#30038=DIRECTION('center_axis',(0.,1.,0.));
#30039=DIRECTION('ref_axis',(1.,0.,0.));
#30040=DIRECTION('center_axis',(0.,1.,0.));
#30041=DIRECTION('ref_axis',(1.,0.,0.));
#30042=DIRECTION('center_axis',(0.,1.,0.));
#30043=DIRECTION('ref_axis',(1.,0.,0.));
#30044=DIRECTION('center_axis',(0.,1.,0.));
#30045=DIRECTION('ref_axis',(1.,0.,0.));
#30046=DIRECTION('center_axis',(0.,-1.,0.));
#30047=DIRECTION('ref_axis',(0.,0.,1.));
#30048=DIRECTION('center_axis',(0.,-1.,0.));
#30049=DIRECTION('ref_axis',(-0.707106781186551,0.,-0.707106781186544));
#30050=DIRECTION('center_axis',(0.,-1.,0.));
#30051=DIRECTION('ref_axis',(-1.,0.,0.));
#30052=DIRECTION('',(0.,-1.,0.));
#30053=DIRECTION('center_axis',(0.,1.,0.));
#30054=DIRECTION('ref_axis',(0.,0.,-1.));
#30055=DIRECTION('',(0.,1.,0.));
#30056=DIRECTION('center_axis',(-1.,4.44089209850062E-15,0.));
#30057=DIRECTION('ref_axis',(0.,0.,-1.));
#30058=DIRECTION('center_axis',(0.,0.,-1.));
#30059=DIRECTION('ref_axis',(-0.707106781186548,-0.707106781186548,0.));
#30060=DIRECTION('center_axis',(0.,0.,1.));
#30061=DIRECTION('ref_axis',(-0.707106781186548,-0.707106781186548,0.));
#30062=DIRECTION('center_axis',(1.,0.,0.));
#30063=DIRECTION('ref_axis',(0.,-0.707106781186549,-0.707106781186546));
#30064=DIRECTION('center_axis',(-1.,-4.44089209850062E-15,0.));
#30065=DIRECTION('ref_axis',(0.,0.,-1.));
#30066=DIRECTION('',(-1.,0.,0.));
#30067=DIRECTION('',(1.,0.,0.));
#30068=DIRECTION('center_axis',(-4.44089209850064E-15,-1.,0.));
#30069=DIRECTION('ref_axis',(0.,0.,-1.));
#30070=DIRECTION('center_axis',(0.,0.,-1.));
#30071=DIRECTION('ref_axis',(0.707106781186547,-0.707106781186548,0.));
#30072=DIRECTION('center_axis',(0.,0.,1.));
#30073=DIRECTION('ref_axis',(0.707106781186547,-0.707106781186548,0.));
#30074=DIRECTION('center_axis',(0.,1.,0.));
#30075=DIRECTION('ref_axis',(0.707106781186551,0.,-0.707106781186544));
#30076=DIRECTION('center_axis',(0.,-1.,0.));
#30077=DIRECTION('ref_axis',(0.,0.,-1.));
#30078=DIRECTION('',(0.,-1.,0.));
#30079=DIRECTION('',(0.,1.,0.));
#30080=DIRECTION('center_axis',(1.,-4.44089209850062E-15,0.));
#30081=DIRECTION('ref_axis',(0.,0.,-1.));
#30082=DIRECTION('center_axis',(0.,0.,-1.));
#30083=DIRECTION('ref_axis',(0.707106781186549,0.707106781186546,0.));
#30084=DIRECTION('center_axis',(0.,0.,1.));
#30085=DIRECTION('ref_axis',(0.707106781186549,0.707106781186546,0.));
#30086=DIRECTION('center_axis',(-1.,0.,0.));
#30087=DIRECTION('ref_axis',(0.,0.707106781186551,-0.707106781186544));
#30088=DIRECTION('center_axis',(1.,4.44089209850062E-15,0.));
#30089=DIRECTION('ref_axis',(0.,0.,-1.));
#30090=DIRECTION('',(1.,0.,0.));
#30091=DIRECTION('',(-1.,0.,0.));
#30092=DIRECTION('center_axis',(0.,0.,-1.));
#30093=DIRECTION('ref_axis',(-0.707106781186546,0.707106781186549,0.));
#30094=DIRECTION('center_axis',(0.,0.,1.));
#30095=DIRECTION('ref_axis',(-0.707106781186546,0.707106781186549,0.));
#30096=DIRECTION('center_axis',(0.,0.,1.));
#30097=DIRECTION('ref_axis',(1.,4.4408920985006E-15,0.));
#30098=DIRECTION('',(0.,0.,1.));
#30099=DIRECTION('center_axis',(0.,0.,1.));
#30100=DIRECTION('ref_axis',(0.707106781186549,0.707106781186546,0.));
#30101=DIRECTION('',(0.,0.,1.));
#30102=DIRECTION('center_axis',(0.,1.,0.));
#30103=DIRECTION('ref_axis',(-1.,0.,0.));
#30104=DIRECTION('',(0.,0.,1.));
#30105=DIRECTION('',(-1.,0.,0.));
#30106=DIRECTION('center_axis',(0.,0.,1.));
#30107=DIRECTION('ref_axis',(-4.4408920985006E-15,1.,0.));
#30108=DIRECTION('',(0.,0.,1.));
#30109=DIRECTION('center_axis',(0.,0.,1.));
#30110=DIRECTION('ref_axis',(-0.707106781186546,0.707106781186549,0.));
#30111=DIRECTION('center_axis',(-1.,0.,0.));
#30112=DIRECTION('ref_axis',(0.,-1.,0.));
#30113=DIRECTION('',(0.,0.,1.));
#30114=DIRECTION('',(0.,-1.,0.));
#30115=DIRECTION('center_axis',(0.,0.,1.));
#30116=DIRECTION('ref_axis',(1.,0.,0.));
#30117=DIRECTION('center_axis',(0.,0.,1.));
#30118=DIRECTION('ref_axis',(1.,0.,0.));
#30119=DIRECTION('center_axis',(0.,0.,1.));
#30120=DIRECTION('ref_axis',(1.,0.,0.));
#30121=DIRECTION('center_axis',(1.,0.,0.));
#30122=DIRECTION('ref_axis',(0.,-0.707106781186549,0.707106781186546));
#30123=DIRECTION('center_axis',(1.,0.,0.));
#30124=DIRECTION('ref_axis',(0.,0.,1.));
#30125=DIRECTION('',(1.,0.,0.));
#30126=DIRECTION('center_axis',(-1.,-4.44089209850062E-15,0.));
#30127=DIRECTION('ref_axis',(4.44089209850062E-15,-1.,0.));
#30128=DIRECTION('',(-1.,0.,0.));
#30129=DIRECTION('center_axis',(-4.44089209850064E-15,-1.,0.));
#30130=DIRECTION('ref_axis',(1.,-4.44089209850064E-15,0.));
#30131=DIRECTION('center_axis',(0.,0.,-1.));
#30132=DIRECTION('ref_axis',(0.707106781186547,-0.707106781186548,0.));
#30133=DIRECTION('center_axis',(0.,0.,1.));
#30134=DIRECTION('ref_axis',(0.707106781186547,-0.707106781186548,0.));
#30135=DIRECTION('center_axis',(0.,1.,0.));
#30136=DIRECTION('ref_axis',(0.707106781186551,0.,0.707106781186544));
#30137=DIRECTION('center_axis',(0.,-1.,0.));
#30138=DIRECTION('ref_axis',(1.,0.,0.));
#30139=DIRECTION('',(0.,-1.,0.));
#30140=DIRECTION('',(0.,1.,0.));
#30141=DIRECTION('center_axis',(1.,-4.44089209850062E-15,0.));
#30142=DIRECTION('ref_axis',(4.44089209850062E-15,1.,0.));
#30143=DIRECTION('center_axis',(0.,0.,-1.));
#30144=DIRECTION('ref_axis',(0.707106781186549,0.707106781186546,0.));
#30145=DIRECTION('center_axis',(-1.,0.,0.));
#30146=DIRECTION('ref_axis',(0.,0.707106781186551,0.707106781186544));
#30147=DIRECTION('center_axis',(1.,4.44089209850062E-15,0.));
#30148=DIRECTION('ref_axis',(-4.44089209850062E-15,1.,0.));
#30149=DIRECTION('',(1.,0.,0.));
#30150=DIRECTION('center_axis',(4.44089209850062E-15,1.,0.));
#30151=DIRECTION('ref_axis',(-1.,4.44089209850062E-15,0.));
#30152=DIRECTION('center_axis',(0.,0.,-1.));
#30153=DIRECTION('ref_axis',(-0.707106781186546,0.707106781186549,0.));
#30154=DIRECTION('center_axis',(0.,-1.,0.));
#30155=DIRECTION('ref_axis',(-0.707106781186551,0.,0.707106781186544));
#30156=DIRECTION('center_axis',(0.,1.,0.));
#30157=DIRECTION('ref_axis',(-1.,0.,0.));
#30158=DIRECTION('',(0.,1.,0.));
#30159=DIRECTION('center_axis',(0.,0.,-1.));
#30160=DIRECTION('ref_axis',(-0.707106781186548,-0.707106781186548,0.));
#30161=DIRECTION('center_axis',(0.,0.,1.));
#30162=DIRECTION('ref_axis',(-0.707106781186548,-0.707106781186548,0.));
#30163=DIRECTION('center_axis',(1.,0.,0.));
#30164=DIRECTION('ref_axis',(0.,1.,0.));
#30165=DIRECTION('',(0.,0.,1.));
#30166=DIRECTION('center_axis',(0.,0.,1.));
#30167=DIRECTION('ref_axis',(2.2204460492503E-15,-1.,0.));
#30168=DIRECTION('',(0.,0.,1.));
#30169=DIRECTION('center_axis',(0.,-1.,0.));
#30170=DIRECTION('ref_axis',(1.,0.,0.));
#30171=DIRECTION('',(0.,0.,1.));
#30172=DIRECTION('center_axis',(0.,0.,1.));
#30173=DIRECTION('ref_axis',(1.,0.,0.));
#30174=DIRECTION('center_axis',(0.,0.,1.));
#30175=DIRECTION('ref_axis',(7.40148683083437E-16,-1.,0.));
#30176=DIRECTION('',(1.,0.,0.));
#30177=DIRECTION('center_axis',(0.,0.,1.));
#30178=DIRECTION('ref_axis',(-1.,-1.11022302462516E-15,0.));
#30179=DIRECTION('',(0.,-1.,0.));
#30180=DIRECTION('center_axis',(0.,0.,1.));
#30181=DIRECTION('ref_axis',(-2.22044604925031E-15,1.,0.));
#30182=DIRECTION('',(-1.,0.,0.));
#30183=DIRECTION('center_axis',(0.,0.,1.));
#30184=DIRECTION('ref_axis',(1.,2.22044604925031E-15,0.));
#30185=DIRECTION('',(0.,1.,0.));
#30186=DIRECTION('center_axis',(0.,0.,-1.));
#30187=DIRECTION('ref_axis',(1.,0.,0.));
#30188=DIRECTION('center_axis',(0.,0.,-1.));
#30189=DIRECTION('ref_axis',(1.,0.,0.));
#30190=DIRECTION('center_axis',(0.,-1.,0.));
#30191=DIRECTION('ref_axis',(-0.707106781186557,0.,0.707106781186538));
#30192=DIRECTION('center_axis',(0.,-1.,0.));
#30193=DIRECTION('ref_axis',(0.,0.,1.));
#30194=DIRECTION('',(0.,-1.,0.));
#30195=DIRECTION('center_axis',(0.,1.,0.));
#30196=DIRECTION('ref_axis',(-1.,0.,0.));
#30197=DIRECTION('',(0.,1.,0.));
#30198=DIRECTION('center_axis',(-1.,0.,0.));
#30199=DIRECTION('ref_axis',(0.,-1.,0.));
#30200=DIRECTION('center_axis',(0.,0.,-1.));
#30201=DIRECTION('ref_axis',(-0.707106781186548,-0.707106781186548,0.));
#30202=DIRECTION('center_axis',(0.,0.,1.));
#30203=DIRECTION('ref_axis',(-0.707106781186547,-0.707106781186547,0.));
#30204=DIRECTION('center_axis',(1.,0.,0.));
#30205=DIRECTION('ref_axis',(0.,-0.707106781186555,0.70710678118654));
#30206=DIRECTION('center_axis',(-1.,0.,0.));
#30207=DIRECTION('ref_axis',(0.,-1.,0.));
#30208=DIRECTION('',(-1.,0.,0.));
#30209=DIRECTION('',(1.,0.,0.));
#30210=DIRECTION('center_axis',(2.22044604925031E-15,-1.,0.));
#30211=DIRECTION('ref_axis',(1.,2.22044604925031E-15,0.));
#30212=DIRECTION('center_axis',(0.,0.,-1.));
#30213=DIRECTION('ref_axis',(0.707106781186548,-0.707106781186548,0.));
#30214=DIRECTION('center_axis',(0.,0.,1.));
#30215=DIRECTION('ref_axis',(0.707106781186548,-0.707106781186548,0.));
#30216=DIRECTION('center_axis',(0.,1.,0.));
#30217=DIRECTION('ref_axis',(0.707106781186555,0.,0.70710678118654));
#30218=DIRECTION('center_axis',(0.,-1.,0.));
#30219=DIRECTION('ref_axis',(1.,0.,0.));
#30220=DIRECTION('',(0.,-1.,0.));
#30221=DIRECTION('',(0.,1.,0.));
#30222=DIRECTION('center_axis',(1.,2.22044604925032E-15,0.));
#30223=DIRECTION('ref_axis',(-2.22044604925032E-15,1.,0.));
#30224=DIRECTION('center_axis',(0.,0.,-1.));
#30225=DIRECTION('ref_axis',(0.707106781186548,0.707106781186548,0.));
#30226=DIRECTION('center_axis',(0.,0.,1.));
#30227=DIRECTION('ref_axis',(0.707106781186548,0.707106781186548,0.));
#30228=DIRECTION('center_axis',(-1.,0.,0.));
#30229=DIRECTION('ref_axis',(0.,0.707106781186555,0.70710678118654));
#30230=DIRECTION('center_axis',(1.,0.,0.));
#30231=DIRECTION('ref_axis',(0.,1.,0.));
#30232=DIRECTION('',(1.,0.,0.));
#30233=DIRECTION('',(-1.,0.,0.));
#30234=DIRECTION('center_axis',(0.,0.,-1.));
#30235=DIRECTION('ref_axis',(-0.707106781186549,0.707106781186546,0.));
#30236=DIRECTION('center_axis',(0.,0.,1.));
#30237=DIRECTION('ref_axis',(-0.707106781186549,0.707106781186546,0.));
#30238=DIRECTION('center_axis',(0.,0.,1.));
#30239=DIRECTION('ref_axis',(-1.48029736616688E-15,-1.,0.));
#30240=DIRECTION('',(0.,0.,1.));
#30241=DIRECTION('center_axis',(0.,0.,-1.));
#30242=DIRECTION('ref_axis',(-1.48029736616688E-15,-1.,0.));
#30243=DIRECTION('',(0.,0.,1.));
#30244=DIRECTION('center_axis',(0.,-1.,0.));
#30245=DIRECTION('ref_axis',(1.,0.,0.));
#30246=DIRECTION('',(0.,0.,1.));
#30247=DIRECTION('',(-1.,0.,0.));
#30248=DIRECTION('center_axis',(0.,0.,1.));
#30249=DIRECTION('ref_axis',(-1.,-1.48029736616687E-15,0.));
#30250=DIRECTION('',(0.,0.,1.));
#30251=DIRECTION('center_axis',(0.,0.,-1.));
#30252=DIRECTION('ref_axis',(-1.,-1.48029736616687E-15,0.));
#30253=DIRECTION('center_axis',(-1.,0.,0.));
#30254=DIRECTION('ref_axis',(0.,-1.,0.));
#30255=DIRECTION('',(0.,0.,1.));
#30256=DIRECTION('',(0.,1.,0.));
#30257=DIRECTION('center_axis',(0.,0.,1.));
#30258=DIRECTION('ref_axis',(1.,0.,0.));
#30259=DIRECTION('center_axis',(0.,0.,-1.));
#30260=DIRECTION('ref_axis',(1.,0.,0.));
#30261=DIRECTION('center_axis',(0.,-1.,0.));
#30262=DIRECTION('ref_axis',(-0.707106781186555,0.,0.70710678118654));
#30263=DIRECTION('center_axis',(0.,-1.,0.));
#30264=DIRECTION('ref_axis',(0.,0.,1.));
#30265=DIRECTION('',(0.,-1.,0.));
#30266=DIRECTION('center_axis',(0.,1.,0.));
#30267=DIRECTION('ref_axis',(-1.,0.,0.));
#30268=DIRECTION('',(0.,1.,0.));
#30269=DIRECTION('center_axis',(-1.,-2.22044604925031E-15,0.));
#30270=DIRECTION('ref_axis',(2.22044604925031E-15,-1.,0.));
#30271=DIRECTION('center_axis',(0.,0.,-1.));
#30272=DIRECTION('ref_axis',(-0.707106781186548,-0.707106781186548,0.));
#30273=DIRECTION('center_axis',(0.,0.,1.));
#30274=DIRECTION('ref_axis',(-0.707106781186548,-0.707106781186548,0.));
#30275=DIRECTION('center_axis',(1.,0.,0.));
#30276=DIRECTION('ref_axis',(0.,-0.707106781186555,0.70710678118654));
#30277=DIRECTION('center_axis',(-1.,0.,0.));
#30278=DIRECTION('ref_axis',(0.,-1.,0.));
#30279=DIRECTION('',(-1.,0.,0.));
#30280=DIRECTION('',(1.,0.,0.));
#30281=DIRECTION('center_axis',(-2.22044604925031E-15,-1.,0.));
#30282=DIRECTION('ref_axis',(1.,-2.22044604925031E-15,0.));
#30283=DIRECTION('center_axis',(0.,0.,-1.));
#30284=DIRECTION('ref_axis',(0.707106781186548,-0.707106781186548,0.));
#30285=DIRECTION('center_axis',(0.,0.,1.));
#30286=DIRECTION('ref_axis',(0.707106781186547,-0.707106781186547,0.));
#30287=DIRECTION('center_axis',(0.,1.,0.));
#30288=DIRECTION('ref_axis',(0.707106781186557,0.,0.707106781186538));
#30289=DIRECTION('center_axis',(0.,-1.,0.));
#30290=DIRECTION('ref_axis',(1.,0.,0.));
#30291=DIRECTION('',(0.,-1.,0.));
#30292=DIRECTION('',(0.,1.,0.));
#30293=DIRECTION('center_axis',(1.,0.,0.));
#30294=DIRECTION('ref_axis',(0.,1.,0.));
#30295=DIRECTION('center_axis',(0.,0.,-1.));
#30296=DIRECTION('ref_axis',(0.707106781186548,0.707106781186547,0.));
#30297=DIRECTION('center_axis',(0.,0.,1.));
#30298=DIRECTION('ref_axis',(0.707106781186548,0.707106781186547,0.));
#30299=DIRECTION('center_axis',(-1.,0.,0.));
#30300=DIRECTION('ref_axis',(0.,0.707106781186555,0.70710678118654));
#30301=DIRECTION('center_axis',(1.,0.,0.));
#30302=DIRECTION('ref_axis',(0.,1.,0.));
#30303=DIRECTION('',(1.,0.,0.));
#30304=DIRECTION('',(-1.,0.,0.));
#30305=DIRECTION('center_axis',(0.,0.,-1.));
#30306=DIRECTION('ref_axis',(-0.707106781186549,0.707106781186546,0.));
#30307=DIRECTION('center_axis',(0.,0.,1.));
#30308=DIRECTION('ref_axis',(-0.707106781186549,0.707106781186546,0.));
#30309=DIRECTION('center_axis',(0.,0.,1.));
#30310=DIRECTION('ref_axis',(0.,-1.,0.));
#30311=DIRECTION('',(0.,0.,1.));
#30312=DIRECTION('center_axis',(0.,0.,-1.));
#30313=DIRECTION('ref_axis',(0.,-1.,0.));
#30314=DIRECTION('',(0.,0.,1.));
#30315=DIRECTION('center_axis',(0.,-1.,0.));
#30316=DIRECTION('ref_axis',(1.,0.,0.));
#30317=DIRECTION('',(0.,0.,1.));
#30318=DIRECTION('',(-1.,0.,0.));
#30319=DIRECTION('center_axis',(0.,0.,1.));
#30320=DIRECTION('ref_axis',(-1.,1.48029736616688E-15,0.));
#30321=DIRECTION('',(0.,0.,1.));
#30322=DIRECTION('center_axis',(0.,0.,-1.));
#30323=DIRECTION('ref_axis',(-1.,1.48029736616688E-15,0.));
#30324=DIRECTION('center_axis',(-1.,0.,0.));
#30325=DIRECTION('ref_axis',(0.,-1.,0.));
#30326=DIRECTION('',(0.,0.,1.));
#30327=DIRECTION('',(0.,1.,0.));
#30328=DIRECTION('center_axis',(0.,0.,1.));
#30329=DIRECTION('ref_axis',(1.,0.,0.));
#30330=DIRECTION('center_axis',(0.,0.,-1.));
#30331=DIRECTION('ref_axis',(1.,0.,0.));
#30332=DIRECTION('center_axis',(0.,1.,0.));
#30333=DIRECTION('ref_axis',(0.,0.,1.));
#30334=DIRECTION('center_axis',(-1.,0.,1.22464679914735E-16));
#30335=DIRECTION('ref_axis',(-1.22464679914735E-16,0.,-1.));
#30336=DIRECTION('center_axis',(0.,1.,0.));
#30337=DIRECTION('ref_axis',(0.,0.,1.));
#30338=DIRECTION('center_axis',(0.,1.,0.));
#30339=DIRECTION('ref_axis',(0.,0.,1.));
#30340=DIRECTION('',(0.,1.,0.));
#30341=DIRECTION('center_axis',(0.,1.,0.));
#30342=DIRECTION('ref_axis',(0.5,0.,0.866025403784439));
#30343=DIRECTION('',(0.,1.,0.));
#30344=DIRECTION('center_axis',(0.,1.,0.));
#30345=DIRECTION('ref_axis',(1.,0.,0.));
#30346=DIRECTION('',(0.,1.,0.));
#30347=DIRECTION('center_axis',(0.,1.,0.));
#30348=DIRECTION('ref_axis',(0.5,0.,0.866025403784439));
#30349=DIRECTION('center_axis',(0.,1.,0.));
#30350=DIRECTION('ref_axis',(0.,0.,1.));
#30351=DIRECTION('center_axis',(0.,-1.,0.));
#30352=DIRECTION('ref_axis',(6.12323399573677E-17,0.,-1.));
#30353=DIRECTION('center_axis',(-1.,0.,1.22464679914735E-16));
#30354=DIRECTION('ref_axis',(-1.22464679914735E-16,0.,-1.));
#30355=DIRECTION('center_axis',(0.,1.,0.));
#30356=DIRECTION('ref_axis',(6.12323399573677E-17,0.,-1.));
#30357=DIRECTION('center_axis',(0.,1.,0.));
#30358=DIRECTION('ref_axis',(0.,0.,1.));
#30359=DIRECTION('',(-0.499999999999999,0.,-0.866025403784439));
#30360=DIRECTION('',(-0.5,0.,0.866025403784439));
#30361=DIRECTION('center_axis',(0.,1.,0.));
#30362=DIRECTION('ref_axis',(-1.1686558153949E-16,0.,-1.));
#30363=DIRECTION('center_axis',(0.,1.,0.));
#30364=DIRECTION('ref_axis',(0.,0.,1.));
#30365=DIRECTION('',(0.,1.,0.));
#30366=DIRECTION('center_axis',(0.,1.,0.));
#30367=DIRECTION('ref_axis',(1.,0.,0.));
#30368=DIRECTION('center_axis',(0.499999999999999,0.,0.866025403784439));
#30369=DIRECTION('ref_axis',(0.612372435695794,-0.707106781186549,-0.353553390593273));
#30370=DIRECTION('',(0.499999999999999,0.,0.866025403784439));
#30371=DIRECTION('center_axis',(0.,-1.,0.));
#30372=DIRECTION('ref_axis',(0.,0.,-1.));
#30373=DIRECTION('center_axis',(0.,-1.,0.));
#30374=DIRECTION('ref_axis',(-1.1686558153949E-16,0.,-1.));
#30375=DIRECTION('center_axis',(0.5,0.,-0.866025403784439));
#30376=DIRECTION('ref_axis',(-0.612372435695795,-0.707106781186548,-0.353553390593273));
#30377=DIRECTION('',(0.5,0.,-0.866025403784439));
#30378=DIRECTION('center_axis',(-0.866025403784439,0.,0.499999999999999));
#30379=DIRECTION('ref_axis',(0.499999999999999,0.,0.866025403784439));
#30380=DIRECTION('',(0.,1.,0.));
#30381=DIRECTION('',(0.499999999999999,0.,0.866025403784439));
#30382=DIRECTION('center_axis',(0.,1.,0.));
#30383=DIRECTION('ref_axis',(1.55820775385987E-16,0.,-1.));
#30384=DIRECTION('',(0.,1.,0.));
#30385=DIRECTION('center_axis',(0.,-1.,0.));
#30386=DIRECTION('ref_axis',(0.5,0.,0.866025403784439));
#30387=DIRECTION('center_axis',(0.866025403784439,0.,0.5));
#30388=DIRECTION('ref_axis',(0.5,0.,-0.866025403784439));
#30389=DIRECTION('',(0.5,0.,-0.866025403784439));
#30390=DIRECTION('center_axis',(-1.,0.,0.));
#30391=DIRECTION('ref_axis',(0.,0.,1.));
#30392=DIRECTION('center_axis',(-7.2886433738689E-15,0.474973683481511,
0.880000000000003));
#30393=DIRECTION('ref_axis',(1.,-1.11022302462515E-15,8.8817841970012E-15));
#30394=DIRECTION('center_axis',(-1.,0.,0.));
#30395=DIRECTION('ref_axis',(0.,1.5907673188659E-15,1.));
#30396=DIRECTION('center_axis',(-1.,0.,0.));
#30397=DIRECTION('ref_axis',(0.,1.5907673188659E-15,1.));
#30398=DIRECTION('center_axis',(0.,-0.474973683481513,0.880000000000002));
#30399=DIRECTION('ref_axis',(0.,-0.880000000000002,-0.474973683481513));
#30400=DIRECTION('center_axis',(1.,0.,0.));
#30401=DIRECTION('ref_axis',(0.,1.5907673188659E-15,1.));
#30402=DIRECTION('center_axis',(-1.02090452894056E-12,0.474973683483218,
0.879999999999082));
#30403=DIRECTION('ref_axis',(0.,-0.879999999999082,0.474973683483219));
#30404=DIRECTION('center_axis',(-1.,0.,0.));
#30405=DIRECTION('ref_axis',(0.,-9.12405358762789E-13,-1.));
#30406=DIRECTION('center_axis',(-5.27326719492196E-16,0.474973683481515,
-0.880000000000001));
#30407=DIRECTION('ref_axis',(0.,0.880000000000001,0.474973683481515));
#30408=DIRECTION('center_axis',(1.,0.,0.));
#30409=DIRECTION('ref_axis',(0.,2.12102309182119E-15,-1.));
#30410=DIRECTION('center_axis',(-1.,0.,0.));
#30411=DIRECTION('ref_axis',(0.,2.12102309182119E-15,-1.));
#30412=DIRECTION('center_axis',(0.,0.,1.));
#30413=DIRECTION('ref_axis',(-5.92118946466753E-15,-1.,0.));
#30414=DIRECTION('',(0.,0.,1.));
#30415=DIRECTION('center_axis',(0.,0.,1.));
#30416=DIRECTION('ref_axis',(0.707106781186548,-0.707106781186547,0.));
#30417=DIRECTION('',(0.,0.,1.));
#30418=DIRECTION('center_axis',(0.,0.,1.));
#30419=DIRECTION('ref_axis',(-5.92118946466753E-15,-1.,0.));
#30420=DIRECTION('',(0.,0.,1.));
#30421=DIRECTION('center_axis',(1.,0.,0.));
#30422=DIRECTION('ref_axis',(0.,1.,0.));
#30423=DIRECTION('',(0.,0.,1.));
#30424=DIRECTION('',(0.,1.,0.));
#30425=DIRECTION('center_axis',(-1.,0.,0.));
#30426=DIRECTION('ref_axis',(0.,0.,-1.));
#30427=DIRECTION('',(-1.,0.,0.));
#30428=DIRECTION('center_axis',(-1.,0.,0.));
#30429=DIRECTION('ref_axis',(0.,0.,-1.));
#30430=DIRECTION('center_axis',(-1.,0.,0.));
#30431=DIRECTION('ref_axis',(0.,0.707106781186544,-0.707106781186551));
#30432=DIRECTION('',(-1.,0.,0.));
#30433=DIRECTION('center_axis',(1.,8.88178419700124E-15,0.));
#30434=DIRECTION('ref_axis',(0.,0.,-1.));
#30435=DIRECTION('',(1.,0.,0.));
#30436=DIRECTION('center_axis',(0.,-1.,0.));
#30437=DIRECTION('ref_axis',(-0.707106781186544,0.,-0.707106781186551));
#30438=DIRECTION('center_axis',(0.,-1.,0.));
#30439=DIRECTION('ref_axis',(-1.,0.,0.));
#30440=DIRECTION('',(0.,-1.,0.));
#30441=DIRECTION('center_axis',(-1.11022302462516E-15,1.,0.));
#30442=DIRECTION('ref_axis',(0.,0.,-1.));
#30443=DIRECTION('',(0.,1.,0.));
#30444=DIRECTION('center_axis',(0.,0.,1.));
#30445=DIRECTION('ref_axis',(1.,0.,0.));
#30446=DIRECTION('center_axis',(-1.,-8.88178419700125E-15,0.));
#30447=DIRECTION('ref_axis',(0.,0.,-1.));
#30448=DIRECTION('center_axis',(0.,0.,-1.));
#30449=DIRECTION('ref_axis',(-0.707106781186545,-0.70710678118655,0.));
#30450=DIRECTION('center_axis',(0.,0.,1.));
#30451=DIRECTION('ref_axis',(-0.707106781186545,-0.70710678118655,0.));
#30452=DIRECTION('center_axis',(1.,0.,0.));
#30453=DIRECTION('ref_axis',(0.,-0.707106781186546,-0.707106781186549));
#30454=DIRECTION('',(-1.,0.,0.));
#30455=DIRECTION('',(1.,0.,0.));
#30456=DIRECTION('center_axis',(0.,0.,1.));
#30457=DIRECTION('ref_axis',(1.,0.,0.));
#30458=DIRECTION('center_axis',(0.,0.,-1.));
#30459=DIRECTION('ref_axis',(-0.707106781186548,0.707106781186548,0.));
#30460=DIRECTION('center_axis',(0.,0.,1.));
#30461=DIRECTION('ref_axis',(-0.707106781186548,0.707106781186548,0.));
#30462=DIRECTION('center_axis',(0.,0.,1.));
#30463=DIRECTION('ref_axis',(-1.,4.44089209850066E-15,0.));
#30464=DIRECTION('',(0.,0.,1.));
#30465=DIRECTION('center_axis',(0.,0.,1.));
#30466=DIRECTION('ref_axis',(-0.707106781186545,-0.70710678118655,0.));
#30467=DIRECTION('',(0.,0.,1.));
#30468=DIRECTION('',(0.,0.,1.));
#30469=DIRECTION('center_axis',(0.,-1.,0.));
#30470=DIRECTION('ref_axis',(1.,0.,0.));
#30471=DIRECTION('',(1.,0.,0.));
#30472=DIRECTION('',(1.,0.,0.));
#30473=DIRECTION('center_axis',(0.,0.,1.));
#30474=DIRECTION('ref_axis',(1.,0.,0.));
#30475=DIRECTION('center_axis',(0.,-1.,0.));
#30476=DIRECTION('ref_axis',(-0.707106781186548,0.,0.707106781186548));
#30477=DIRECTION('center_axis',(0.,-1.,0.));
#30478=DIRECTION('ref_axis',(0.,0.,1.));
#30479=DIRECTION('',(0.,-1.,0.));
#30480=DIRECTION('center_axis',(-1.11022302462516E-15,1.,0.));
#30481=DIRECTION('ref_axis',(-1.,-1.11022302462516E-15,0.));
#30482=DIRECTION('',(0.,1.,0.));
#30483=DIRECTION('center_axis',(0.,0.,1.));
#30484=DIRECTION('ref_axis',(1.,0.,0.));
#30485=DIRECTION('center_axis',(-1.,-8.88178419700125E-15,0.));
#30486=DIRECTION('ref_axis',(8.88178419700125E-15,-1.,0.));
#30487=DIRECTION('center_axis',(0.,0.,-1.));
#30488=DIRECTION('ref_axis',(-0.707106781186545,-0.70710678118655,0.));
#30489=DIRECTION('center_axis',(1.,0.,0.));
#30490=DIRECTION('ref_axis',(0.,-0.707106781186549,0.707106781186546));
#30491=DIRECTION('center_axis',(-1.,0.,0.));
#30492=DIRECTION('ref_axis',(0.,-1.,0.));
#30493=DIRECTION('',(-1.,0.,0.));
#30494=DIRECTION('center_axis',(0.,0.,1.));
#30495=DIRECTION('ref_axis',(1.,0.,0.));
#30496=DIRECTION('center_axis',(4.4408920985006E-15,-1.,0.));
#30497=DIRECTION('ref_axis',(1.,4.4408920985006E-15,0.));
#30498=DIRECTION('center_axis',(0.,0.,-1.));
#30499=DIRECTION('ref_axis',(0.707106781186548,-0.707106781186547,0.));
#30500=DIRECTION('center_axis',(0.,1.,0.));
#30501=DIRECTION('ref_axis',(0.707106781186548,0.,0.707106781186548));
#30502=DIRECTION('center_axis',(0.,-1.,0.));
#30503=DIRECTION('ref_axis',(1.,0.,0.));
#30504=DIRECTION('',(0.,-1.,0.));
#30505=DIRECTION('center_axis',(0.,0.,1.));
#30506=DIRECTION('ref_axis',(1.,0.,0.));
#30507=DIRECTION('center_axis',(1.,0.,0.));
#30508=DIRECTION('ref_axis',(0.,1.,0.));
#30509=DIRECTION('center_axis',(0.,0.,-1.));
#30510=DIRECTION('ref_axis',(0.707106781186548,0.707106781186548,0.));
#30511=DIRECTION('center_axis',(0.,0.,1.));
#30512=DIRECTION('ref_axis',(0.707106781186548,0.707106781186548,0.));
#30513=DIRECTION('center_axis',(-1.,0.,0.));
#30514=DIRECTION('ref_axis',(0.,0.707106781186548,0.707106781186548));
#30515=DIRECTION('center_axis',(1.,8.88178419700124E-15,0.));
#30516=DIRECTION('ref_axis',(-8.88178419700124E-15,1.,0.));
#30517=DIRECTION('',(1.,0.,0.));
#30518=DIRECTION('',(-1.,0.,0.));
#30519=DIRECTION('center_axis',(0.,0.,1.));
#30520=DIRECTION('ref_axis',(1.,0.,0.));
#30521=DIRECTION('center_axis',(0.,0.,-1.));
#30522=DIRECTION('ref_axis',(-0.707106781186548,0.707106781186548,0.));
#30523=DIRECTION('center_axis',(0.,0.,1.));
#30524=DIRECTION('ref_axis',(-0.707106781186548,0.707106781186548,0.));
#30525=DIRECTION('center_axis',(-1.,0.,0.));
#30526=DIRECTION('ref_axis',(0.,-1.,0.));
#30527=DIRECTION('',(0.,0.,1.));
#30528=DIRECTION('center_axis',(-1.,0.,0.));
#30529=DIRECTION('ref_axis',(0.,-1.32563943238825E-15,1.));
#30530=DIRECTION('center_axis',(0.,0.,1.));
#30531=DIRECTION('ref_axis',(1.,0.,0.));
#30532=DIRECTION('center_axis',(0.,0.,-1.));
#30533=DIRECTION('ref_axis',(0.,1.,0.));
#30534=DIRECTION('',(1.,0.,0.));
#30535=DIRECTION('center_axis',(0.,0.,-1.));
#30536=DIRECTION('ref_axis',(1.,-4.44089209850064E-15,0.));
#30537=DIRECTION('',(0.,-1.,0.));
#30538=DIRECTION('center_axis',(0.,0.,-1.));
#30539=DIRECTION('ref_axis',(2.96059473233376E-15,1.,0.));
#30540=DIRECTION('',(1.,0.,0.));
#30541=DIRECTION('center_axis',(0.,0.,-1.));
#30542=DIRECTION('ref_axis',(1.,-1.48029736616687E-15,0.));
#30543=DIRECTION('',(0.,-1.,0.));
#30544=DIRECTION('center_axis',(0.,0.,-1.));
#30545=DIRECTION('ref_axis',(1.,0.,0.));
#30546=DIRECTION('center_axis',(1.,0.,0.));
#30547=DIRECTION('ref_axis',(0.,5.1364535115188E-16,1.));
#30548=DIRECTION('center_axis',(0.,-0.47497368348152,0.879999999999998));
#30549=DIRECTION('ref_axis',(-1.,0.,0.));
#30550=DIRECTION('center_axis',(1.,0.,0.));
#30551=DIRECTION('ref_axis',(0.,-1.32563943238825E-15,1.));
#30552=DIRECTION('center_axis',(1.,0.,0.));
#30553=DIRECTION('ref_axis',(0.,-1.32563943238825E-15,1.));
#30554=DIRECTION('center_axis',(0.,0.474973683481518,0.88));
#30555=DIRECTION('ref_axis',(0.,0.88,-0.474973683481518));
#30556=DIRECTION('center_axis',(1.02248650909906E-12,-0.474973683483223,
0.879999999999079));
#30557=DIRECTION('ref_axis',(0.,0.879999999999079,0.474973683483223));
#30558=DIRECTION('center_axis',(1.,0.,0.));
#30559=DIRECTION('ref_axis',(0.,0.,-1.));
#30560=DIRECTION('center_axis',(0.,-0.474973683481516,-0.88));
#30561=DIRECTION('ref_axis',(0.,-0.88,0.474973683481516));
#30562=DIRECTION('center_axis',(-1.,0.,0.));
#30563=DIRECTION('ref_axis',(0.,-1.0605115459106E-15,-1.));
#30564=DIRECTION('center_axis',(1.,0.,0.));
#30565=DIRECTION('ref_axis',(0.,-1.0605115459106E-15,-1.));
#30566=DIRECTION('center_axis',(0.,0.,1.));
#30567=DIRECTION('ref_axis',(2.96059473233376E-15,1.,0.));
#30568=DIRECTION('',(0.,0.,1.));
#30569=DIRECTION('',(0.,0.,1.));
#30570=DIRECTION('center_axis',(1.,0.,0.));
#30571=DIRECTION('ref_axis',(0.,0.,-1.));
#30572=DIRECTION('',(1.,0.,0.));
#30573=DIRECTION('center_axis',(1.,0.,0.));
#30574=DIRECTION('ref_axis',(0.,0.,-1.));
#30575=DIRECTION('center_axis',(0.,0.,-1.));
#30576=DIRECTION('ref_axis',(1.,0.,0.));
#30577=DIRECTION('',(0.,0.,-1.));
#30578=DIRECTION('center_axis',(0.,0.,-1.));
#30579=DIRECTION('ref_axis',(1.,0.,0.));
#30580=DIRECTION('',(0.,0.,-1.));
#30581=DIRECTION('center_axis',(0.,0.,-1.));
#30582=DIRECTION('ref_axis',(1.,0.,0.));
#30583=DIRECTION('',(0.,0.,-1.));
#30584=DIRECTION('center_axis',(0.,0.,-1.));
#30585=DIRECTION('ref_axis',(1.,0.,0.));
#30586=DIRECTION('center_axis',(0.,0.,1.));
#30587=DIRECTION('ref_axis',(1.,0.,0.));
#30588=DIRECTION('center_axis',(0.,0.,-1.));
#30589=DIRECTION('ref_axis',(1.,0.,0.));
#30590=DIRECTION('',(0.,0.,-1.));
#30591=DIRECTION('center_axis',(0.,0.,-1.));
#30592=DIRECTION('ref_axis',(1.,0.,0.));
#30593=DIRECTION('center_axis',(0.,0.,1.));
#30594=DIRECTION('ref_axis',(1.,0.,0.));
#30595=DIRECTION('center_axis',(0.,0.,-1.));
#30596=DIRECTION('ref_axis',(1.,0.,0.));
#30597=DIRECTION('',(0.,0.,-1.));
#30598=DIRECTION('center_axis',(0.,0.,-1.));
#30599=DIRECTION('ref_axis',(1.,0.,0.));
#30600=DIRECTION('center_axis',(0.,0.,1.));
#30601=DIRECTION('ref_axis',(1.,0.,0.));
#30602=DIRECTION('center_axis',(1.,0.,0.));
#30603=DIRECTION('ref_axis',(0.,0.,-1.));
#30604=DIRECTION('center_axis',(-1.,0.,0.));
#30605=DIRECTION('ref_axis',(0.,-1.,0.));
#30606=DIRECTION('center_axis',(1.,0.,0.));
#30607=DIRECTION('ref_axis',(0.,0.,-1.));
#30608=DIRECTION('center_axis',(1.,0.,0.));
#30609=DIRECTION('ref_axis',(0.,1.,0.));
#30610=DIRECTION('',(0.,1.,0.));
#30611=DIRECTION('',(0.,0.,1.));
#30612=DIRECTION('center_axis',(0.,-1.,0.));
#30613=DIRECTION('ref_axis',(1.,0.,0.));
#30614=DIRECTION('',(0.,-1.,0.));
#30615=DIRECTION('center_axis',(0.,-1.,0.));
#30616=DIRECTION('ref_axis',(1.,0.,0.));
#30617=DIRECTION('center_axis',(0.,1.,0.));
#30618=DIRECTION('ref_axis',(1.,0.,0.));
#30619=DIRECTION('center_axis',(0.,-1.,0.));
#30620=DIRECTION('ref_axis',(1.,0.,0.));
#30621=DIRECTION('',(0.,-1.,0.));
#30622=DIRECTION('center_axis',(0.,-1.,0.));
#30623=DIRECTION('ref_axis',(1.,0.,0.));
#30624=DIRECTION('center_axis',(0.,1.,0.));
#30625=DIRECTION('ref_axis',(1.,0.,0.));
#30626=DIRECTION('center_axis',(0.,-1.,0.));
#30627=DIRECTION('ref_axis',(1.,0.,0.));
#30628=DIRECTION('',(0.,-1.,0.));
#30629=DIRECTION('center_axis',(0.,-1.,0.));
#30630=DIRECTION('ref_axis',(1.,0.,0.));
#30631=DIRECTION('center_axis',(0.,1.,0.));
#30632=DIRECTION('ref_axis',(1.,0.,0.));
#30633=DIRECTION('center_axis',(0.,-1.,0.));
#30634=DIRECTION('ref_axis',(1.,0.,0.));
#30635=DIRECTION('',(0.,-1.,0.));
#30636=DIRECTION('center_axis',(0.,-1.,0.));
#30637=DIRECTION('ref_axis',(1.,0.,0.));
#30638=DIRECTION('center_axis',(0.,1.,0.));
#30639=DIRECTION('ref_axis',(1.,0.,0.));
#30640=DIRECTION('center_axis',(0.,1.,0.));
#30641=DIRECTION('ref_axis',(1.,0.,0.));
#30642=DIRECTION('',(0.,1.,0.));
#30643=DIRECTION('center_axis',(0.,1.,0.));
#30644=DIRECTION('ref_axis',(1.,0.,0.));
#30645=DIRECTION('center_axis',(0.,1.,0.));
#30646=DIRECTION('ref_axis',(1.,0.,0.));
#30647=DIRECTION('center_axis',(0.,1.,0.));
#30648=DIRECTION('ref_axis',(1.,0.,0.));
#30649=DIRECTION('',(0.,1.,0.));
#30650=DIRECTION('center_axis',(0.,1.,0.));
#30651=DIRECTION('ref_axis',(1.,0.,0.));
#30652=DIRECTION('center_axis',(0.,1.,0.));
#30653=DIRECTION('ref_axis',(1.,0.,0.));
#30654=DIRECTION('center_axis',(0.,1.,0.));
#30655=DIRECTION('ref_axis',(1.,0.,0.));
#30656=DIRECTION('',(0.,1.,0.));
#30657=DIRECTION('center_axis',(0.,1.,0.));
#30658=DIRECTION('ref_axis',(1.,0.,0.));
#30659=DIRECTION('center_axis',(0.,1.,0.));
#30660=DIRECTION('ref_axis',(1.,0.,0.));
#30661=DIRECTION('center_axis',(0.,1.,0.));
#30662=DIRECTION('ref_axis',(1.,0.,0.));
#30663=DIRECTION('',(0.,1.,0.));
#30664=DIRECTION('center_axis',(0.,1.,0.));
#30665=DIRECTION('ref_axis',(1.,0.,0.));
#30666=DIRECTION('center_axis',(0.,1.,0.));
#30667=DIRECTION('ref_axis',(1.,0.,0.));
#30668=DIRECTION('center_axis',(0.,1.,0.));
#30669=DIRECTION('ref_axis',(1.,0.,0.));
#30670=DIRECTION('',(0.,1.,0.));
#30671=DIRECTION('center_axis',(0.,1.,0.));
#30672=DIRECTION('ref_axis',(1.,0.,0.));
#30673=DIRECTION('center_axis',(0.,1.,0.));
#30674=DIRECTION('ref_axis',(1.,0.,0.));
#30675=DIRECTION('center_axis',(0.,1.,0.));
#30676=DIRECTION('ref_axis',(1.,0.,0.));
#30677=DIRECTION('',(0.,1.,0.));
#30678=DIRECTION('center_axis',(0.,1.,0.));
#30679=DIRECTION('ref_axis',(1.,0.,0.));
#30680=DIRECTION('center_axis',(0.,1.,0.));
#30681=DIRECTION('ref_axis',(1.,0.,0.));
#30682=DIRECTION('center_axis',(0.,1.,0.));
#30683=DIRECTION('ref_axis',(1.,0.,0.));
#30684=DIRECTION('',(0.,1.,0.));
#30685=DIRECTION('center_axis',(0.,1.,0.));
#30686=DIRECTION('ref_axis',(1.,0.,0.));
#30687=DIRECTION('center_axis',(0.,1.,0.));
#30688=DIRECTION('ref_axis',(1.,0.,0.));
#30689=DIRECTION('center_axis',(0.,1.,0.));
#30690=DIRECTION('ref_axis',(1.,0.,0.));
#30691=DIRECTION('',(0.,1.,0.));
#30692=DIRECTION('center_axis',(0.,1.,0.));
#30693=DIRECTION('ref_axis',(1.,0.,0.));
#30694=DIRECTION('center_axis',(0.,1.,0.));
#30695=DIRECTION('ref_axis',(1.,0.,0.));
#30696=DIRECTION('center_axis',(0.,1.,0.));
#30697=DIRECTION('ref_axis',(1.,0.,0.));
#30698=DIRECTION('center_axis',(0.,1.,0.));
#30699=DIRECTION('ref_axis',(0.,0.,1.));
#30700=DIRECTION('center_axis',(0.,1.,0.));
#30701=DIRECTION('ref_axis',(1.,0.,0.));
#30702=DIRECTION('center_axis',(0.,1.,0.));
#30703=DIRECTION('ref_axis',(0.,0.,1.));
#30704=DIRECTION('',(0.,1.,0.));
#30705=DIRECTION('center_axis',(0.,0.,1.));
#30706=DIRECTION('ref_axis',(2.96059473233376E-15,1.,0.));
#30707=DIRECTION('',(0.,0.,1.));
#30708=DIRECTION('center_axis',(0.,1.,0.));
#30709=DIRECTION('ref_axis',(-1.,0.,0.));
#30710=DIRECTION('',(0.,0.,1.));
#30711=DIRECTION('center_axis',(0.,0.,1.));
#30712=DIRECTION('ref_axis',(1.,-1.48029736616687E-15,0.));
#30713=DIRECTION('',(0.,0.,1.));
#30714=DIRECTION('center_axis',(1.,0.,0.));
#30715=DIRECTION('ref_axis',(0.,1.,0.));
#30716=DIRECTION('center_axis',(0.,0.,1.));
#30717=DIRECTION('ref_axis',(0.,1.,0.));
#30718=DIRECTION('',(0.,0.,1.));
#30719=DIRECTION('center_axis',(0.,1.,0.));
#30720=DIRECTION('ref_axis',(-1.,0.,0.));
#30721=DIRECTION('',(0.,0.,1.));
#30722=DIRECTION('center_axis',(0.,0.,1.));
#30723=DIRECTION('ref_axis',(1.,-4.44089209850064E-15,0.));
#30724=DIRECTION('',(0.,0.,1.));
#30725=DIRECTION('center_axis',(1.,0.,0.));
#30726=DIRECTION('ref_axis',(0.,1.,0.));
#30727=DIRECTION('center_axis',(0.,0.,1.));
#30728=DIRECTION('ref_axis',(-1.,-4.44089209850061E-15,0.));
#30729=DIRECTION('center_axis',(0.,0.,1.));
#30730=DIRECTION('ref_axis',(7.40148683083437E-16,-1.,0.));
#30731=DIRECTION('',(0.,0.,1.));
#30732=DIRECTION('',(0.,0.,1.));
#30733=DIRECTION('center_axis',(0.,-1.,0.));
#30734=DIRECTION('ref_axis',(1.,0.,0.));
#30735=DIRECTION('',(0.,0.,1.));
#30736=DIRECTION('center_axis',(0.,0.,1.));
#30737=DIRECTION('ref_axis',(-1.,-1.11022302462516E-15,0.));
#30738=DIRECTION('',(0.,0.,1.));
#30739=DIRECTION('center_axis',(-1.,0.,0.));
#30740=DIRECTION('ref_axis',(0.,-1.,0.));
#30741=DIRECTION('',(0.,0.,1.));
#30742=DIRECTION('center_axis',(0.,0.,1.));
#30743=DIRECTION('ref_axis',(-2.22044604925031E-15,1.,0.));
#30744=DIRECTION('',(0.,0.,1.));
#30745=DIRECTION('center_axis',(0.,1.,0.));
#30746=DIRECTION('ref_axis',(-1.,0.,0.));
#30747=DIRECTION('',(0.,0.,1.));
#30748=DIRECTION('center_axis',(0.,0.,1.));
#30749=DIRECTION('ref_axis',(1.,2.22044604925031E-15,0.));
#30750=DIRECTION('',(0.,0.,1.));
#30751=DIRECTION('center_axis',(1.,0.,0.));
#30752=DIRECTION('ref_axis',(0.,1.,0.));
#30753=DIRECTION('center_axis',(0.,0.,1.));
#30754=DIRECTION('ref_axis',(1.,0.,0.));
#30755=DIRECTION('',(1.,0.,0.));
#30756=DIRECTION('center_axis',(0.,0.,1.));
#30757=DIRECTION('ref_axis',(1.,-2.96059473233376E-15,0.));
#30758=DIRECTION('center_axis',(0.,1.,0.));
#30759=DIRECTION('ref_axis',(-1.,0.,0.));
#30760=DIRECTION('',(0.,0.,1.));
#30761=DIRECTION('center_axis',(0.,0.,1.));
#30762=DIRECTION('ref_axis',(1.,-2.96059473233376E-15,0.));
#37376=CARTESIAN_POINT('',(0.,0.,0.));
#37377=CARTESIAN_POINT('Origin',(0.,46.,0.));
#37378=CARTESIAN_POINT('',(76.9075363365802,47.,50.));
#37379=CARTESIAN_POINT('',(77.2269383052313,46.,50.));
#37380=CARTESIAN_POINT('Ctrl Pts',(77.2269383052313,46.,50.));
#37381=CARTESIAN_POINT('Ctrl Pts',(77.2269383052313,46.2329198319017,50.));
#37382=CARTESIAN_POINT('Ctrl Pts',(77.1653607660612,46.5055561829699,50.));
#37383=CARTESIAN_POINT('Ctrl Pts',(77.0254295449815,46.8110812445886,50.));
#37384=CARTESIAN_POINT('Ctrl Pts',(76.9710438766786,46.9077781744567,50.));
#37385=CARTESIAN_POINT('Ctrl Pts',(76.9075363365807,46.9999999999992,50.));
#37386=CARTESIAN_POINT('',(-1.12667505521556E-14,46.,-92.));
#37387=CARTESIAN_POINT('Origin',(0.,46.,0.));
#37388=CARTESIAN_POINT('',(1.10218211923262E-14,48.,-90.));
#37389=CARTESIAN_POINT('Origin',(-1.10218211923262E-14,46.,-90.));
#37390=CARTESIAN_POINT('Origin',(0.,48.,0.));
#37391=CARTESIAN_POINT('',(-77.0527954329529,45.9999999996096,50.2679491919803));
#37392=CARTESIAN_POINT('Origin',(0.,46.,0.));
#37393=CARTESIAN_POINT('',(-75.5696311051099,47.,52.));
#37394=CARTESIAN_POINT('Ctrl Pts',(-75.5696311051099,47.,52.));
#37395=CARTESIAN_POINT('Ctrl Pts',(-75.5700201424603,47.,51.999434626749));
#37396=CARTESIAN_POINT('Ctrl Pts',(-75.570409287503,46.9999997602648,51.9988693275745));
#37397=CARTESIAN_POINT('Ctrl Pts',(-75.5720130884468,46.9999977855239,51.9965404836838));
#37398=CARTESIAN_POINT('Ctrl Pts',(-75.5732286826425,46.9999939579146,51.994777587995));
#37399=CARTESIAN_POINT('Ctrl Pts',(-75.5765121990975,46.999977349045,51.9900217507738));
#37400=CARTESIAN_POINT('Ctrl Pts',(-75.5785820799728,46.9999601799197,51.9870301822449));
#37401=CARTESIAN_POINT('Ctrl Pts',(-75.5887090256785,46.9998436332333,51.972425137894));
#37402=CARTESIAN_POINT('Ctrl Pts',(-75.5968078544418,46.9996500011623,51.9608415795779));
#37403=CARTESIAN_POINT('Ctrl Pts',(-75.6621771593858,46.997297854563,51.8681016030327));
#37404=CARTESIAN_POINT('Ctrl Pts',(-75.7215624039282,46.9903378312819,51.7885093232287));
#37405=CARTESIAN_POINT('Ctrl Pts',(-75.9151544327206,46.9541413446516,51.540847638037));
#37406=CARTESIAN_POINT('Ctrl Pts',(-76.0564163554542,46.9079528904244,51.3776580388172));
#37407=CARTESIAN_POINT('Ctrl Pts',(-76.4041124085987,46.7468902883554,50.9947551668813));
#37408=CARTESIAN_POINT('Ctrl Pts',(-76.6102052861138,46.6079794397508,50.7845705159268));
#37409=CARTESIAN_POINT('Ctrl Pts',(-76.8970989561146,46.3036584894847,50.4719619095292));
#37410=CARTESIAN_POINT('Ctrl Pts',(-76.9933165723146,46.1579139502934,50.3591208541419));
#37411=CARTESIAN_POINT('Ctrl Pts',(-77.0527954326587,46.0000000000002,50.2679491924312));
#37412=CARTESIAN_POINT('Origin',(0.,47.,0.));
#37413=CARTESIAN_POINT('Origin',(0.,24.,0.));
#37414=CARTESIAN_POINT('',(77.2269383052313,2.,50.));
#37415=CARTESIAN_POINT('',(77.2269383052313,24.,50.));
#37416=CARTESIAN_POINT('',(43.1452924241198,2.,-81.2556689815375));
#37417=CARTESIAN_POINT('Origin',(0.,2.,0.));
#37418=CARTESIAN_POINT('',(39.,2.,-83.3246662159531));
#37419=CARTESIAN_POINT('Origin',(0.,2.,0.));
#37420=CARTESIAN_POINT('',(45.,8.,-80.2433797892387));
#37421=CARTESIAN_POINT('Ctrl Pts',(39.,2.,-83.3246662159531));
#37422=CARTESIAN_POINT('Ctrl Pts',(39.7682076868648,2.,-82.965107622462));
#37423=CARTESIAN_POINT('Ctrl Pts',(40.5861518890197,2.1556365878507,-82.5680240102596));
#37424=CARTESIAN_POINT('Ctrl Pts',(42.0962197288883,2.79558990411642,-81.8084506557891));
#37425=CARTESIAN_POINT('Ctrl Pts',(42.7886063451273,3.27986145745522,-81.4464457673431));
#37426=CARTESIAN_POINT('Ctrl Pts',(43.825446345948,4.36512188826461,-80.8927389962394));
#37427=CARTESIAN_POINT('Ctrl Pts',(44.2621585987635,5.01413618672815,-80.6534196360022));
#37428=CARTESIAN_POINT('Ctrl Pts',(44.8497980701861,6.45547542071794,-80.3281295509505));
#37429=CARTESIAN_POINT('Ctrl Pts',(45.,7.24837120717834,-80.2433797892387));
#37430=CARTESIAN_POINT('Ctrl Pts',(45.,8.00000000000001,-80.2433797892387));
#37431=CARTESIAN_POINT('',(45.,36.,-80.2433797892387));
#37432=CARTESIAN_POINT('',(45.,24.,-80.2433797892387));
#37433=CARTESIAN_POINT('',(39.,42.,-83.3246662159531));
#37434=CARTESIAN_POINT('Ctrl Pts',(45.,36.,-80.2433797892387));
#37435=CARTESIAN_POINT('Ctrl Pts',(45.,36.7516287928217,-80.2433797892387));
#37436=CARTESIAN_POINT('Ctrl Pts',(44.8497980701861,37.5445245792821,-80.3281295509505));
#37437=CARTESIAN_POINT('Ctrl Pts',(44.2621585987635,38.9858638132718,-80.6534196360022));
#37438=CARTESIAN_POINT('Ctrl Pts',(43.8254463459479,39.6348781117354,-80.8927389962394));
#37439=CARTESIAN_POINT('Ctrl Pts',(42.7886063451273,40.7201385425448,-81.4464457673431));
#37440=CARTESIAN_POINT('Ctrl Pts',(42.0962197288883,41.2044100958836,-81.8084506557891));
#37441=CARTESIAN_POINT('Ctrl Pts',(40.5861518890197,41.8443634121493,-82.5680240102596));
#37442=CARTESIAN_POINT('Ctrl Pts',(39.7682076868648,42.,-82.965107622462));
#37443=CARTESIAN_POINT('Ctrl Pts',(39.,42.,-83.3246662159531));
#37444=CARTESIAN_POINT('',(-39.,42.,-83.3246662159531));
#37445=CARTESIAN_POINT('Origin',(0.,42.,0.));
#37446=CARTESIAN_POINT('',(-45.,36.,-80.2433797892387));
#37447=CARTESIAN_POINT('Ctrl Pts',(-39.,42.,-83.3246662159531));
#37448=CARTESIAN_POINT('Ctrl Pts',(-39.7682076868648,42.,-82.965107622462));
#37449=CARTESIAN_POINT('Ctrl Pts',(-40.5861518890197,41.8443634121493,-82.5680240102596));
#37450=CARTESIAN_POINT('Ctrl Pts',(-42.0962197288883,41.2044100958836,-81.8084506557891));
#37451=CARTESIAN_POINT('Ctrl Pts',(-42.7886063451273,40.7201385425448,-81.4464457673431));
#37452=CARTESIAN_POINT('Ctrl Pts',(-43.8254463459479,39.6348781117354,-80.8927389962394));
#37453=CARTESIAN_POINT('Ctrl Pts',(-44.2621585987635,38.9858638132719,-80.6534196360022));
#37454=CARTESIAN_POINT('Ctrl Pts',(-44.8497980701861,37.5445245792821,-80.3281295509504));
#37455=CARTESIAN_POINT('Ctrl Pts',(-45.,36.7516287928217,-80.2433797892387));
#37456=CARTESIAN_POINT('Ctrl Pts',(-45.,36.,-80.2433797892387));
#37457=CARTESIAN_POINT('',(-45.,8.,-80.2433797892387));
#37458=CARTESIAN_POINT('',(-45.,24.,-80.2433797892387));
#37459=CARTESIAN_POINT('',(-39.,2.,-83.3246662159531));
#37460=CARTESIAN_POINT('Ctrl Pts',(-45.,8.00000000000001,-80.2433797892387));
#37461=CARTESIAN_POINT('Ctrl Pts',(-45.,7.24837120717834,-80.2433797892387));
#37462=CARTESIAN_POINT('Ctrl Pts',(-44.8497980701861,6.45547542071794,-80.3281295509505));
#37463=CARTESIAN_POINT('Ctrl Pts',(-44.2621585987635,5.01413618672815,-80.6534196360022));
#37464=CARTESIAN_POINT('Ctrl Pts',(-43.8254463459479,4.36512188826461,-80.8927389962394));
#37465=CARTESIAN_POINT('Ctrl Pts',(-42.7886063451273,3.27986145745522,-81.4464457673431));
#37466=CARTESIAN_POINT('Ctrl Pts',(-42.0962197288883,2.79558990411642,-81.8084506557891));
#37467=CARTESIAN_POINT('Ctrl Pts',(-40.5861518890197,2.1556365878507,-82.5680240102596));
#37468=CARTESIAN_POINT('Ctrl Pts',(-39.7682076868648,2.,-82.965107622462));
#37469=CARTESIAN_POINT('Ctrl Pts',(-39.,2.,-83.3246662159531));
#37470=CARTESIAN_POINT('',(-75.8946638440411,2.,52.));
#37471=CARTESIAN_POINT('Origin',(0.,2.,0.));
#37472=CARTESIAN_POINT('',(-77.2269383052313,4.,50.));
#37473=CARTESIAN_POINT('Ctrl Pts',(-75.8946638440411,2.,52.));
#37474=CARTESIAN_POINT('Ctrl Pts',(-76.0674525460939,2.,51.7478126834933));
#37475=CARTESIAN_POINT('Ctrl Pts',(-76.2523381437454,2.05028979164384,51.4749989417307));
#37476=CARTESIAN_POINT('Ctrl Pts',(-76.5947876563318,2.26685914288403,50.9640372439704));
#37477=CARTESIAN_POINT('Ctrl Pts',(-76.7523839779586,2.43326063418965,50.7259626978856));
#37478=CARTESIAN_POINT('Ctrl Pts',(-76.9789947123575,2.80370034162261,50.3812329006827));
#37479=CARTESIAN_POINT('Ctrl Pts',(-77.0709575562652,3.01592897574302,50.2402273896437));
#37480=CARTESIAN_POINT('Ctrl Pts',(-77.1949935065466,3.48961682480797,50.0494348028582));
#37481=CARTESIAN_POINT('Ctrl Pts',(-77.2269383052313,3.75125143583077,50.));
#37482=CARTESIAN_POINT('Ctrl Pts',(-77.2269383052313,4.,50.));
#37483=CARTESIAN_POINT('',(-77.2269383052313,45.,50.));
#37484=CARTESIAN_POINT('',(-77.2269383052313,24.,50.));
#37485=CARTESIAN_POINT('Ctrl Pts',(-77.2269383052313,45.,50.));
#37486=CARTESIAN_POINT('Ctrl Pts',(-77.2269383052313,45.2487485641692,50.));
#37487=CARTESIAN_POINT('Ctrl Pts',(-77.1949935065466,45.510383175192,50.0494348028582));
#37488=CARTESIAN_POINT('Ctrl Pts',(-77.109956799136,45.8351346277627,50.1802386008037));
#37489=CARTESIAN_POINT('Ctrl Pts',(-77.082972874874,45.919880120673,50.2216919585661));
#37490=CARTESIAN_POINT('Ctrl Pts',(-77.0527954328532,45.9999999994838,50.2679491921331));
#37491=CARTESIAN_POINT('Origin',(0.,48.,0.));
#37492=CARTESIAN_POINT('',(-46.0621933088198,48.,-41.0121933088198));
#37493=CARTESIAN_POINT('Origin',(-41.0121933088198,48.,-41.0121933088198));
#37494=CARTESIAN_POINT('',(-46.0621933088198,48.,41.0121933088198));
#37495=CARTESIAN_POINT('Origin',(-41.0121933088198,48.,41.0121933088198));
#37496=CARTESIAN_POINT('',(35.9621933088198,48.,41.0121933088198));
#37497=CARTESIAN_POINT('Origin',(41.0121933088198,48.,41.0121933088198));
#37498=CARTESIAN_POINT('',(35.9621933088197,48.,-41.0121933088198));
#37499=CARTESIAN_POINT('Origin',(41.0121933088197,48.,-41.0121933088198));
#37500=CARTESIAN_POINT('',(1.59204083889156E-15,48.,-13.));
#37501=CARTESIAN_POINT('Origin',(0.,48.,0.));
#37502=CARTESIAN_POINT('Origin',(0.,2.,0.));
#37503=CARTESIAN_POINT('',(42.207351284465,1.66533453693773E-15,-79.4892413949823));
#37504=CARTESIAN_POINT('Origin',(42.207351284465,2.,-79.4892413949823));
#37505=CARTESIAN_POINT('Origin',(0.,1.66533453693773E-15,0.));
#37506=CARTESIAN_POINT('Origin',(0.,2.,0.));
#37507=CARTESIAN_POINT('Origin',(0.,2.,0.));
#37508=CARTESIAN_POINT('Origin',(0.,0.,91.));
#37509=CARTESIAN_POINT('',(26.3300414539374,0.,-75.7581216659255));
#37510=CARTESIAN_POINT('Origin',(31.3800414539374,0.,-75.7581216659255));
#37511=CARTESIAN_POINT('',(-80.8081216659255,0.,-31.3800414539373));
#37512=CARTESIAN_POINT('Origin',(-75.7581216659255,0.,-31.3800414539373));
#37513=CARTESIAN_POINT('',(-80.8081216659255,0.,31.3800414539374));
#37514=CARTESIAN_POINT('Origin',(-75.7581216659255,0.,31.3800414539374));
#37515=CARTESIAN_POINT('',(26.3300414539374,0.,75.7581216659255));
#37516=CARTESIAN_POINT('Origin',(31.3800414539374,0.,75.7581216659255));
#37517=CARTESIAN_POINT('',(-36.4300414539374,0.,75.7581216659255));
#37518=CARTESIAN_POINT('Origin',(-31.3800414539374,0.,75.7581216659255));
#37519=CARTESIAN_POINT('',(70.7081216659255,0.,31.3800414539374));
#37520=CARTESIAN_POINT('Origin',(75.7581216659255,0.,31.3800414539374));
#37521=CARTESIAN_POINT('',(-36.4300414539373,0.,-75.7581216659255));
#37522=CARTESIAN_POINT('Origin',(-31.3800414539373,0.,-75.7581216659255));
#37523=CARTESIAN_POINT('',(70.7081216659255,0.,-31.3800414539373));
#37524=CARTESIAN_POINT('Origin',(75.7581216659255,0.,-31.3800414539373));
#37525=CARTESIAN_POINT('',(8.84194988984389E-15,0.,-72.2));
#37526=CARTESIAN_POINT('Origin',(0.,0.,0.));
#37527=CARTESIAN_POINT('Origin',(-73.,28.,-138.));
#37528=CARTESIAN_POINT('',(-75.,41.,-138.));
#37529=CARTESIAN_POINT('',(-73.,41.,-140.));
#37530=CARTESIAN_POINT('Origin',(-73.,41.,-138.));
#37531=CARTESIAN_POINT('',(-73.,-11.,-140.));
#37532=CARTESIAN_POINT('',(-73.,28.,-140.));
#37533=CARTESIAN_POINT('',(-75.,-11.,-138.));
#37534=CARTESIAN_POINT('Origin',(-73.,-11.,-138.));
#37535=CARTESIAN_POINT('',(-75.,28.,-138.));
#37536=CARTESIAN_POINT('Ctrl Pts',(-73.,-11.,-140.));
#37537=CARTESIAN_POINT('Ctrl Pts',(-73.,-13.,-140.));
#37538=CARTESIAN_POINT('Ctrl Pts',(-71.,-13.,-140.));
#37539=CARTESIAN_POINT('Ctrl Pts',(-75.,-11.,-140.));
#37540=CARTESIAN_POINT('Ctrl Pts',(-75.,-15.,-140.));
#37541=CARTESIAN_POINT('Ctrl Pts',(-71.,-15.,-140.));
#37542=CARTESIAN_POINT('Ctrl Pts',(-75.,-11.,-138.));
#37543=CARTESIAN_POINT('Ctrl Pts',(-75.,-15.,-138.));
#37544=CARTESIAN_POINT('Ctrl Pts',(-71.,-15.,-138.));
#37545=CARTESIAN_POINT('',(-71.,-13.,-140.));
#37546=CARTESIAN_POINT('',(-71.,-15.,-138.));
#37547=CARTESIAN_POINT('Origin',(-71.,-13.,-138.));
#37548=CARTESIAN_POINT('Origin',(-71.,-11.,-138.));
#37549=CARTESIAN_POINT('Origin',(-71.,-11.,-140.));
#37550=CARTESIAN_POINT('Origin',(-35.5,-13.,-138.));
#37551=CARTESIAN_POINT('',(71.,-13.,-140.));
#37552=CARTESIAN_POINT('',(71.,-15.,-138.));
#37553=CARTESIAN_POINT('Origin',(71.,-13.,-138.));
#37554=CARTESIAN_POINT('',(-35.5,-15.,-138.));
#37555=CARTESIAN_POINT('',(-35.5,-13.,-140.));
#37556=CARTESIAN_POINT('Ctrl Pts',(71.,-13.,-140.));
#37557=CARTESIAN_POINT('Ctrl Pts',(73.,-13.,-140.));
#37558=CARTESIAN_POINT('Ctrl Pts',(73.,-11.,-140.));
#37559=CARTESIAN_POINT('Ctrl Pts',(71.,-15.,-140.));
#37560=CARTESIAN_POINT('Ctrl Pts',(75.,-15.,-140.));
#37561=CARTESIAN_POINT('Ctrl Pts',(75.,-11.,-140.));
#37562=CARTESIAN_POINT('Ctrl Pts',(71.,-15.,-138.));
#37563=CARTESIAN_POINT('Ctrl Pts',(75.,-15.,-138.));
#37564=CARTESIAN_POINT('Ctrl Pts',(75.,-11.,-138.));
#37565=CARTESIAN_POINT('',(73.,-11.,-140.));
#37566=CARTESIAN_POINT('',(75.,-11.,-138.));
#37567=CARTESIAN_POINT('Origin',(73.,-11.,-138.));
#37568=CARTESIAN_POINT('Origin',(71.,-11.,-138.));
#37569=CARTESIAN_POINT('Origin',(71.,-11.,-140.));
#37570=CARTESIAN_POINT('Origin',(73.,2.,-138.));
#37571=CARTESIAN_POINT('',(73.,41.,-140.));
#37572=CARTESIAN_POINT('',(75.,41.,-138.));
#37573=CARTESIAN_POINT('Origin',(73.,41.,-138.));
#37574=CARTESIAN_POINT('',(75.,2.,-138.));
#37575=CARTESIAN_POINT('',(73.,2.,-140.));
#37576=CARTESIAN_POINT('Ctrl Pts',(73.,41.,-140.));
#37577=CARTESIAN_POINT('Ctrl Pts',(73.,43.,-140.));
#37578=CARTESIAN_POINT('Ctrl Pts',(71.,43.,-140.));
#37579=CARTESIAN_POINT('Ctrl Pts',(75.,41.,-140.));
#37580=CARTESIAN_POINT('Ctrl Pts',(75.,45.,-140.));
#37581=CARTESIAN_POINT('Ctrl Pts',(71.,45.,-140.));
#37582=CARTESIAN_POINT('Ctrl Pts',(75.,41.,-138.));
#37583=CARTESIAN_POINT('Ctrl Pts',(75.,45.,-138.));
#37584=CARTESIAN_POINT('Ctrl Pts',(71.,45.,-138.));
#37585=CARTESIAN_POINT('',(71.,43.,-140.));
#37586=CARTESIAN_POINT('',(71.,45.,-138.));
#37587=CARTESIAN_POINT('Origin',(71.,43.,-138.));
#37588=CARTESIAN_POINT('Origin',(71.,41.,-138.));
#37589=CARTESIAN_POINT('Origin',(71.,41.,-140.));
#37590=CARTESIAN_POINT('Origin',(35.5,43.,-138.));
#37591=CARTESIAN_POINT('',(-71.,43.,-140.));
#37592=CARTESIAN_POINT('',(-71.,45.,-138.));
#37593=CARTESIAN_POINT('Origin',(-71.,43.,-138.));
#37594=CARTESIAN_POINT('',(35.5,45.,-138.));
#37595=CARTESIAN_POINT('',(35.5,43.,-140.));
#37596=CARTESIAN_POINT('Ctrl Pts',(-71.,43.,-140.));
#37597=CARTESIAN_POINT('Ctrl Pts',(-73.,43.,-140.));
#37598=CARTESIAN_POINT('Ctrl Pts',(-73.,41.,-140.));
#37599=CARTESIAN_POINT('Ctrl Pts',(-71.,45.,-140.));
#37600=CARTESIAN_POINT('Ctrl Pts',(-75.,45.,-140.));
#37601=CARTESIAN_POINT('Ctrl Pts',(-75.,41.,-140.));
#37602=CARTESIAN_POINT('Ctrl Pts',(-71.,45.,-138.));
#37603=CARTESIAN_POINT('Ctrl Pts',(-75.,45.,-138.));
#37604=CARTESIAN_POINT('Ctrl Pts',(-75.,41.,-138.));
#37605=CARTESIAN_POINT('Origin',(-71.,41.,-138.));
#37606=CARTESIAN_POINT('Origin',(-71.,41.,-140.));
#37607=CARTESIAN_POINT('Origin',(71.,41.,-140.));
#37608=CARTESIAN_POINT('',(71.,45.,-127.));
#37609=CARTESIAN_POINT('',(71.,45.,-140.));
#37610=CARTESIAN_POINT('',(75.,41.,-127.));
#37611=CARTESIAN_POINT('Origin',(71.,41.,-127.));
#37612=CARTESIAN_POINT('',(75.,41.,-140.));
#37613=CARTESIAN_POINT('Origin',(71.,45.,-140.));
#37614=CARTESIAN_POINT('',(-71.,45.,-127.));
#37615=CARTESIAN_POINT('',(-71.,45.,-140.));
#37616=CARTESIAN_POINT('',(35.5,45.,-127.));
#37617=CARTESIAN_POINT('Origin',(-71.,41.,-140.));
#37618=CARTESIAN_POINT('',(-75.,41.,-127.));
#37619=CARTESIAN_POINT('',(-75.,41.,-140.));
#37620=CARTESIAN_POINT('Origin',(-71.,41.,-127.));
#37621=CARTESIAN_POINT('Origin',(-75.,41.,-140.));
#37622=CARTESIAN_POINT('',(-75.,-11.,-127.));
#37623=CARTESIAN_POINT('',(-75.,-11.,-140.));
#37624=CARTESIAN_POINT('',(-75.,28.,-127.));
#37625=CARTESIAN_POINT('Origin',(0.,15.,-140.));
#37626=CARTESIAN_POINT('',(53.,15.,-140.));
#37627=CARTESIAN_POINT('Origin',(60.,15.,-140.));
#37628=CARTESIAN_POINT('',(-67.,15.,-140.));
#37629=CARTESIAN_POINT('Origin',(-60.,15.,-140.));
#37630=CARTESIAN_POINT('Origin',(-35.5,-13.,-127.));
#37631=CARTESIAN_POINT('',(-71.,-13.,-125.));
#37632=CARTESIAN_POINT('',(-71.,-15.,-127.));
#37633=CARTESIAN_POINT('Origin',(-71.,-13.,-127.));
#37634=CARTESIAN_POINT('',(71.,-15.,-127.));
#37635=CARTESIAN_POINT('',(-35.5,-15.,-127.));
#37636=CARTESIAN_POINT('',(71.,-13.,-125.));
#37637=CARTESIAN_POINT('Origin',(71.,-13.,-127.));
#37638=CARTESIAN_POINT('',(-35.5,-13.,-125.));
#37639=CARTESIAN_POINT('Ctrl Pts',(71.,-15.,-127.));
#37640=CARTESIAN_POINT('Ctrl Pts',(75.,-15.,-127.));
#37641=CARTESIAN_POINT('Ctrl Pts',(75.,-11.,-127.));
#37642=CARTESIAN_POINT('Ctrl Pts',(71.,-15.,-125.));
#37643=CARTESIAN_POINT('Ctrl Pts',(75.,-15.,-125.));
#37644=CARTESIAN_POINT('Ctrl Pts',(75.,-11.,-125.));
#37645=CARTESIAN_POINT('Ctrl Pts',(71.,-13.,-125.));
#37646=CARTESIAN_POINT('Ctrl Pts',(73.,-13.,-125.));
#37647=CARTESIAN_POINT('Ctrl Pts',(73.,-11.,-125.));
#37648=CARTESIAN_POINT('',(75.,-11.,-127.));
#37649=CARTESIAN_POINT('',(73.,-11.,-125.));
#37650=CARTESIAN_POINT('Origin',(73.,-11.,-127.));
#37651=CARTESIAN_POINT('Origin',(71.,-11.,-125.));
#37652=CARTESIAN_POINT('Origin',(71.,-11.,-127.));
#37653=CARTESIAN_POINT('Origin',(73.,2.,-127.));
#37654=CARTESIAN_POINT('',(73.,41.,-125.));
#37655=CARTESIAN_POINT('Origin',(73.,41.,-127.));
#37656=CARTESIAN_POINT('',(73.,2.,-125.));
#37657=CARTESIAN_POINT('',(75.,2.,-127.));
#37658=CARTESIAN_POINT('Ctrl Pts',(75.,41.,-127.));
#37659=CARTESIAN_POINT('Ctrl Pts',(75.,45.,-127.));
#37660=CARTESIAN_POINT('Ctrl Pts',(71.,45.,-127.));
#37661=CARTESIAN_POINT('Ctrl Pts',(75.,41.,-125.));
#37662=CARTESIAN_POINT('Ctrl Pts',(75.,45.,-125.));
#37663=CARTESIAN_POINT('Ctrl Pts',(71.,45.,-125.));
#37664=CARTESIAN_POINT('Ctrl Pts',(73.,41.,-125.));
#37665=CARTESIAN_POINT('Ctrl Pts',(73.,43.,-125.));
#37666=CARTESIAN_POINT('Ctrl Pts',(71.,43.,-125.));
#37667=CARTESIAN_POINT('',(71.,43.,-125.));
#37668=CARTESIAN_POINT('Origin',(71.,43.,-127.));
#37669=CARTESIAN_POINT('Origin',(71.,41.,-125.));
#37670=CARTESIAN_POINT('Origin',(35.5,43.,-127.));
#37671=CARTESIAN_POINT('',(-71.,43.,-125.));
#37672=CARTESIAN_POINT('Origin',(-71.,43.,-127.));
#37673=CARTESIAN_POINT('',(35.5,43.,-125.));
#37674=CARTESIAN_POINT('Ctrl Pts',(-71.,45.,-127.));
#37675=CARTESIAN_POINT('Ctrl Pts',(-75.,45.,-127.));
#37676=CARTESIAN_POINT('Ctrl Pts',(-75.,41.,-127.));
#37677=CARTESIAN_POINT('Ctrl Pts',(-71.,45.,-125.));
#37678=CARTESIAN_POINT('Ctrl Pts',(-75.,45.,-125.));
#37679=CARTESIAN_POINT('Ctrl Pts',(-75.,41.,-125.));
#37680=CARTESIAN_POINT('Ctrl Pts',(-71.,43.,-125.));
#37681=CARTESIAN_POINT('Ctrl Pts',(-73.,43.,-125.));
#37682=CARTESIAN_POINT('Ctrl Pts',(-73.,41.,-125.));
#37683=CARTESIAN_POINT('',(-73.,41.,-125.));
#37684=CARTESIAN_POINT('Origin',(-73.,41.,-127.));
#37685=CARTESIAN_POINT('Origin',(-71.,41.,-125.));
#37686=CARTESIAN_POINT('Origin',(-73.,28.,-127.));
#37687=CARTESIAN_POINT('',(-73.,-11.,-125.));
#37688=CARTESIAN_POINT('Origin',(-73.,-11.,-127.));
#37689=CARTESIAN_POINT('',(-73.,28.,-125.));
#37690=CARTESIAN_POINT('Ctrl Pts',(-75.,-11.,-127.));
#37691=CARTESIAN_POINT('Ctrl Pts',(-75.,-15.,-127.));
#37692=CARTESIAN_POINT('Ctrl Pts',(-71.,-15.,-127.));
#37693=CARTESIAN_POINT('Ctrl Pts',(-75.,-11.,-125.));
#37694=CARTESIAN_POINT('Ctrl Pts',(-75.,-15.,-125.));
#37695=CARTESIAN_POINT('Ctrl Pts',(-71.,-15.,-125.));
#37696=CARTESIAN_POINT('Ctrl Pts',(-73.,-11.,-125.));
#37697=CARTESIAN_POINT('Ctrl Pts',(-73.,-13.,-125.));
#37698=CARTESIAN_POINT('Ctrl Pts',(-71.,-13.,-125.));
#37699=CARTESIAN_POINT('Origin',(-71.,-11.,-125.));
#37700=CARTESIAN_POINT('Origin',(-71.,-11.,-127.));
#37701=CARTESIAN_POINT('Origin',(75.,-11.,-140.));
#37702=CARTESIAN_POINT('',(75.,-11.,-140.));
#37703=CARTESIAN_POINT('Origin',(71.,-11.,-140.));
#37704=CARTESIAN_POINT('',(71.,-15.,-140.));
#37705=CARTESIAN_POINT('Origin',(-71.,-15.,-140.));
#37706=CARTESIAN_POINT('',(-71.,-15.,-140.));
#37707=CARTESIAN_POINT('Origin',(0.,15.,-125.));
#37708=CARTESIAN_POINT('',(39.,2.,-125.));
#37709=CARTESIAN_POINT('',(45.,8.,-125.));
#37710=CARTESIAN_POINT('Origin',(39.,8.00000000000001,-125.));
#37711=CARTESIAN_POINT('',(-39.,2.,-125.));
#37712=CARTESIAN_POINT('',(-39.,2.,-125.));
#37713=CARTESIAN_POINT('',(-45.,8.,-125.));
#37714=CARTESIAN_POINT('Origin',(-39.,8.00000000000001,-125.));
#37715=CARTESIAN_POINT('',(-45.,36.,-125.));
#37716=CARTESIAN_POINT('',(-45.,36.,-125.));
#37717=CARTESIAN_POINT('',(-39.,42.,-125.));
#37718=CARTESIAN_POINT('Origin',(-39.,36.,-125.));
#37719=CARTESIAN_POINT('',(39.,42.,-125.));
#37720=CARTESIAN_POINT('',(39.,42.,-125.));
#37721=CARTESIAN_POINT('',(45.,36.,-125.));
#37722=CARTESIAN_POINT('Origin',(39.,36.,-125.));
#37723=CARTESIAN_POINT('',(45.,8.,-125.));
#37724=CARTESIAN_POINT('',(53.,15.,-125.));
#37725=CARTESIAN_POINT('Origin',(60.,15.,-125.));
#37726=CARTESIAN_POINT('',(-67.,15.,-125.));
#37727=CARTESIAN_POINT('Origin',(-60.,15.,-125.));
#37728=CARTESIAN_POINT('Origin',(-52.,27.5,112.));
#37729=CARTESIAN_POINT('',(-52.,30.5,114.));
#37730=CARTESIAN_POINT('',(-54.,30.5,112.));
#37731=CARTESIAN_POINT('Origin',(-52.,30.5,112.));
#37732=CARTESIAN_POINT('',(-54.,18.5,112.));
#37733=CARTESIAN_POINT('',(-54.,27.5,112.));
#37734=CARTESIAN_POINT('',(-52.,18.5,114.));
#37735=CARTESIAN_POINT('Origin',(-52.,18.5,112.));
#37736=CARTESIAN_POINT('',(-52.,27.5,114.));
#37737=CARTESIAN_POINT('Ctrl Pts',(-54.,18.5,112.));
#37738=CARTESIAN_POINT('Ctrl Pts',(-54.,15.5,112.));
#37739=CARTESIAN_POINT('Ctrl Pts',(-51.,15.5,112.));
#37740=CARTESIAN_POINT('Ctrl Pts',(-54.,18.5,114.));
#37741=CARTESIAN_POINT('Ctrl Pts',(-54.,15.5,114.));
#37742=CARTESIAN_POINT('Ctrl Pts',(-51.,15.5,114.));
#37743=CARTESIAN_POINT('Ctrl Pts',(-52.,18.5,114.));
#37744=CARTESIAN_POINT('Ctrl Pts',(-52.,17.5,114.));
#37745=CARTESIAN_POINT('Ctrl Pts',(-51.,17.5,114.));
#37746=CARTESIAN_POINT('',(-51.,15.5,112.));
#37747=CARTESIAN_POINT('',(-51.,17.5,114.));
#37748=CARTESIAN_POINT('Origin',(-51.,17.5,112.));
#37749=CARTESIAN_POINT('Origin',(-51.,18.5,114.));
#37750=CARTESIAN_POINT('Origin',(-51.,18.5,112.));
#37751=CARTESIAN_POINT('Origin',(-48.,17.5,112.));
#37752=CARTESIAN_POINT('',(-39.,15.5,112.));
#37753=CARTESIAN_POINT('',(-39.,17.5,114.));
#37754=CARTESIAN_POINT('Origin',(-39.,17.5,112.));
#37755=CARTESIAN_POINT('',(-48.,17.5,114.));
#37756=CARTESIAN_POINT('',(-48.,15.5,112.));
#37757=CARTESIAN_POINT('Ctrl Pts',(-39.,15.5,112.));
#37758=CARTESIAN_POINT('Ctrl Pts',(-36.,15.5,112.));
#37759=CARTESIAN_POINT('Ctrl Pts',(-36.,18.5,112.));
#37760=CARTESIAN_POINT('Ctrl Pts',(-39.,15.5,114.));
#37761=CARTESIAN_POINT('Ctrl Pts',(-36.,15.5,114.));
#37762=CARTESIAN_POINT('Ctrl Pts',(-36.,18.5,114.));
#37763=CARTESIAN_POINT('Ctrl Pts',(-39.,17.5,114.));
#37764=CARTESIAN_POINT('Ctrl Pts',(-38.,17.5,114.));
#37765=CARTESIAN_POINT('Ctrl Pts',(-38.,18.5,114.));
#37766=CARTESIAN_POINT('',(-36.,18.5,112.));
#37767=CARTESIAN_POINT('',(-38.,18.5,114.));
#37768=CARTESIAN_POINT('Origin',(-38.,18.5,112.));
#37769=CARTESIAN_POINT('Origin',(-39.,18.5,114.));
#37770=CARTESIAN_POINT('Origin',(-39.,18.5,112.));
#37771=CARTESIAN_POINT('Origin',(-38.,21.5,112.));
#37772=CARTESIAN_POINT('',(-36.,30.5,112.));
#37773=CARTESIAN_POINT('',(-38.,30.5,114.));
#37774=CARTESIAN_POINT('Origin',(-38.,30.5,112.));
#37775=CARTESIAN_POINT('',(-38.,21.5,114.));
#37776=CARTESIAN_POINT('',(-36.,21.5,112.));
#37777=CARTESIAN_POINT('Ctrl Pts',(-36.,30.5,112.));
#37778=CARTESIAN_POINT('Ctrl Pts',(-36.,33.5,112.));
#37779=CARTESIAN_POINT('Ctrl Pts',(-39.,33.5,112.));
#37780=CARTESIAN_POINT('Ctrl Pts',(-36.,30.5,114.));
#37781=CARTESIAN_POINT('Ctrl Pts',(-36.,33.5,114.));
#37782=CARTESIAN_POINT('Ctrl Pts',(-39.,33.5,114.));
#37783=CARTESIAN_POINT('Ctrl Pts',(-38.,30.5,114.));
#37784=CARTESIAN_POINT('Ctrl Pts',(-38.,31.5,114.));
#37785=CARTESIAN_POINT('Ctrl Pts',(-39.,31.5,114.));
#37786=CARTESIAN_POINT('',(-39.,33.5,112.));
#37787=CARTESIAN_POINT('',(-39.,31.5,114.));
#37788=CARTESIAN_POINT('Origin',(-39.,31.5,112.));
#37789=CARTESIAN_POINT('Origin',(-39.,30.5,114.));
#37790=CARTESIAN_POINT('Origin',(-39.,30.5,112.));
#37791=CARTESIAN_POINT('Origin',(-42.,31.5,112.));
#37792=CARTESIAN_POINT('',(-51.,33.5,112.));
#37793=CARTESIAN_POINT('',(-51.,31.5,114.));
#37794=CARTESIAN_POINT('Origin',(-51.,31.5,112.));
#37795=CARTESIAN_POINT('',(-42.,31.5,114.));
#37796=CARTESIAN_POINT('',(-42.,33.5,112.));
#37797=CARTESIAN_POINT('Ctrl Pts',(-51.,33.5,112.));
#37798=CARTESIAN_POINT('Ctrl Pts',(-54.,33.5,112.));
#37799=CARTESIAN_POINT('Ctrl Pts',(-54.,30.5,112.));
#37800=CARTESIAN_POINT('Ctrl Pts',(-51.,33.5,114.));
#37801=CARTESIAN_POINT('Ctrl Pts',(-54.,33.5,114.));
#37802=CARTESIAN_POINT('Ctrl Pts',(-54.,30.5,114.));
#37803=CARTESIAN_POINT('Ctrl Pts',(-51.,31.5,114.));
#37804=CARTESIAN_POINT('Ctrl Pts',(-52.,31.5,114.));
#37805=CARTESIAN_POINT('Ctrl Pts',(-52.,30.5,114.));
#37806=CARTESIAN_POINT('Origin',(-51.,30.5,114.));
#37807=CARTESIAN_POINT('Origin',(-51.,30.5,112.));
#37808=CARTESIAN_POINT('Origin',(-39.,18.5,110.));
#37809=CARTESIAN_POINT('',(-39.,15.5,110.));
#37810=CARTESIAN_POINT('',(-39.,15.5,110.));
#37811=CARTESIAN_POINT('',(-36.,18.5,110.));
#37812=CARTESIAN_POINT('Origin',(-39.,18.5,110.));
#37813=CARTESIAN_POINT('',(-36.,18.5,110.));
#37814=CARTESIAN_POINT('Origin',(-51.,15.5,110.));
#37815=CARTESIAN_POINT('',(-51.,15.5,110.));
#37816=CARTESIAN_POINT('',(-51.,15.5,110.));
#37817=CARTESIAN_POINT('',(-25.5,15.5,110.));
#37818=CARTESIAN_POINT('Origin',(-51.,18.5,110.));
#37819=CARTESIAN_POINT('',(-54.,18.5,110.));
#37820=CARTESIAN_POINT('',(-54.,18.5,110.));
#37821=CARTESIAN_POINT('Origin',(-51.,18.5,110.));
#37822=CARTESIAN_POINT('Origin',(-54.,30.5,110.));
#37823=CARTESIAN_POINT('',(-54.,30.5,110.));
#37824=CARTESIAN_POINT('',(-54.,30.5,110.));
#37825=CARTESIAN_POINT('',(-54.,27.5,110.));
#37826=CARTESIAN_POINT('Origin',(-45.,24.5,114.));
#37827=CARTESIAN_POINT('',(-51.9,24.5,114.));
#37828=CARTESIAN_POINT('Origin',(-45.,24.5,114.));
#37829=CARTESIAN_POINT('Origin',(38.,27.5,112.));
#37830=CARTESIAN_POINT('',(38.,30.5,114.));
#37831=CARTESIAN_POINT('',(36.,30.5,112.));
#37832=CARTESIAN_POINT('Origin',(38.,30.5,112.));
#37833=CARTESIAN_POINT('',(36.,18.5,112.));
#37834=CARTESIAN_POINT('',(36.,27.5,112.));
#37835=CARTESIAN_POINT('',(38.,18.5,114.));
#37836=CARTESIAN_POINT('Origin',(38.,18.5,112.));
#37837=CARTESIAN_POINT('',(38.,27.5,114.));
#37838=CARTESIAN_POINT('Ctrl Pts',(36.,18.5,112.));
#37839=CARTESIAN_POINT('Ctrl Pts',(36.,15.5,112.));
#37840=CARTESIAN_POINT('Ctrl Pts',(39.,15.5,112.));
#37841=CARTESIAN_POINT('Ctrl Pts',(36.,18.5,114.));
#37842=CARTESIAN_POINT('Ctrl Pts',(36.,15.5,114.));
#37843=CARTESIAN_POINT('Ctrl Pts',(39.,15.5,114.));
#37844=CARTESIAN_POINT('Ctrl Pts',(38.,18.5,114.));
#37845=CARTESIAN_POINT('Ctrl Pts',(38.,17.5,114.));
#37846=CARTESIAN_POINT('Ctrl Pts',(39.,17.5,114.));
#37847=CARTESIAN_POINT('',(39.,15.5,112.));
#37848=CARTESIAN_POINT('',(39.,17.5,114.));
#37849=CARTESIAN_POINT('Origin',(39.,17.5,112.));
#37850=CARTESIAN_POINT('Origin',(39.,18.5,114.));
#37851=CARTESIAN_POINT('Origin',(39.,18.5,112.));
#37852=CARTESIAN_POINT('Origin',(42.,17.5,112.));
#37853=CARTESIAN_POINT('',(51.,15.5,112.));
#37854=CARTESIAN_POINT('',(51.,17.5,114.));
#37855=CARTESIAN_POINT('Origin',(51.,17.5,112.));
#37856=CARTESIAN_POINT('',(42.,17.5,114.));
#37857=CARTESIAN_POINT('',(42.,15.5,112.));
#37858=CARTESIAN_POINT('Ctrl Pts',(51.,15.5,112.));
#37859=CARTESIAN_POINT('Ctrl Pts',(54.,15.5,112.));
#37860=CARTESIAN_POINT('Ctrl Pts',(54.,18.5,112.));
#37861=CARTESIAN_POINT('Ctrl Pts',(51.,15.5,114.));
#37862=CARTESIAN_POINT('Ctrl Pts',(54.,15.5,114.));
#37863=CARTESIAN_POINT('Ctrl Pts',(54.,18.5,114.));
#37864=CARTESIAN_POINT('Ctrl Pts',(51.,17.5,114.));
#37865=CARTESIAN_POINT('Ctrl Pts',(52.,17.5,114.));
#37866=CARTESIAN_POINT('Ctrl Pts',(52.,18.5,114.));
#37867=CARTESIAN_POINT('',(54.,18.5,112.));
#37868=CARTESIAN_POINT('',(52.,18.5,114.));
#37869=CARTESIAN_POINT('Origin',(52.,18.5,112.));
#37870=CARTESIAN_POINT('Origin',(51.,18.5,114.));
#37871=CARTESIAN_POINT('Origin',(51.,18.5,112.));
#37872=CARTESIAN_POINT('Origin',(52.,21.5,112.));
#37873=CARTESIAN_POINT('',(54.,30.5,112.));
#37874=CARTESIAN_POINT('',(52.,30.5,114.));
#37875=CARTESIAN_POINT('Origin',(52.,30.5,112.));
#37876=CARTESIAN_POINT('',(52.,21.5,114.));
#37877=CARTESIAN_POINT('',(54.,21.5,112.));
#37878=CARTESIAN_POINT('Ctrl Pts',(54.,30.5,112.));
#37879=CARTESIAN_POINT('Ctrl Pts',(54.,33.5,112.));
#37880=CARTESIAN_POINT('Ctrl Pts',(51.,33.5,112.));
#37881=CARTESIAN_POINT('Ctrl Pts',(54.,30.5,114.));
#37882=CARTESIAN_POINT('Ctrl Pts',(54.,33.5,114.));
#37883=CARTESIAN_POINT('Ctrl Pts',(51.,33.5,114.));
#37884=CARTESIAN_POINT('Ctrl Pts',(52.,30.5,114.));
#37885=CARTESIAN_POINT('Ctrl Pts',(52.,31.5,114.));
#37886=CARTESIAN_POINT('Ctrl Pts',(51.,31.5,114.));
#37887=CARTESIAN_POINT('',(51.,33.5,112.));
#37888=CARTESIAN_POINT('',(51.,31.5,114.));
#37889=CARTESIAN_POINT('Origin',(51.,31.5,112.));
#37890=CARTESIAN_POINT('Origin',(51.,30.5,114.));
#37891=CARTESIAN_POINT('Origin',(51.,30.5,112.));
#37892=CARTESIAN_POINT('Origin',(48.,31.5,112.));
#37893=CARTESIAN_POINT('',(39.,33.5,112.));
#37894=CARTESIAN_POINT('',(39.,31.5,114.));
#37895=CARTESIAN_POINT('Origin',(39.,31.5,112.));
#37896=CARTESIAN_POINT('',(48.,31.5,114.));
#37897=CARTESIAN_POINT('',(48.,33.5,112.));
#37898=CARTESIAN_POINT('Ctrl Pts',(39.,33.5,112.));
#37899=CARTESIAN_POINT('Ctrl Pts',(36.,33.5,112.));
#37900=CARTESIAN_POINT('Ctrl Pts',(36.,30.5,112.));
#37901=CARTESIAN_POINT('Ctrl Pts',(39.,33.5,114.));
#37902=CARTESIAN_POINT('Ctrl Pts',(36.,33.5,114.));
#37903=CARTESIAN_POINT('Ctrl Pts',(36.,30.5,114.));
#37904=CARTESIAN_POINT('Ctrl Pts',(39.,31.5,114.));
#37905=CARTESIAN_POINT('Ctrl Pts',(38.,31.5,114.));
#37906=CARTESIAN_POINT('Ctrl Pts',(38.,30.5,114.));
#37907=CARTESIAN_POINT('Origin',(39.,30.5,114.));
#37908=CARTESIAN_POINT('Origin',(39.,30.5,112.));
#37909=CARTESIAN_POINT('Origin',(51.,18.5,110.));
#37910=CARTESIAN_POINT('',(51.,15.5,110.));
#37911=CARTESIAN_POINT('',(51.,15.5,110.));
#37912=CARTESIAN_POINT('',(54.,18.5,110.));
#37913=CARTESIAN_POINT('Origin',(51.,18.5,110.));
#37914=CARTESIAN_POINT('',(54.,18.5,110.));
#37915=CARTESIAN_POINT('Origin',(39.,15.5,110.));
#37916=CARTESIAN_POINT('',(39.,15.5,110.));
#37917=CARTESIAN_POINT('',(39.,15.5,110.));
#37918=CARTESIAN_POINT('',(19.5,15.5,110.));
#37919=CARTESIAN_POINT('Origin',(39.,18.5,110.));
#37920=CARTESIAN_POINT('',(36.,18.5,110.));
#37921=CARTESIAN_POINT('',(36.,18.5,110.));
#37922=CARTESIAN_POINT('Origin',(39.,18.5,110.));
#37923=CARTESIAN_POINT('Origin',(36.,30.5,110.));
#37924=CARTESIAN_POINT('',(36.,30.5,110.));
#37925=CARTESIAN_POINT('',(36.,30.5,110.));
#37926=CARTESIAN_POINT('',(36.,27.5,110.));
#37927=CARTESIAN_POINT('Origin',(45.,24.5,114.));
#37928=CARTESIAN_POINT('',(38.1,24.5,114.));
#37929=CARTESIAN_POINT('Origin',(45.,24.5,114.));
#37930=CARTESIAN_POINT('Origin',(0.,2.,0.));
#37931=CARTESIAN_POINT('',(-8.59702053001442E-15,2.,-70.2));
#37932=CARTESIAN_POINT('Origin',(-8.84194988984389E-15,2.,-72.2));
#37933=CARTESIAN_POINT('Origin',(0.,2.,0.));
#37934=CARTESIAN_POINT('Origin',(0.,2.45,0.));
#37935=CARTESIAN_POINT('',(-8.59702053001442E-15,9.,-70.2));
#37936=CARTESIAN_POINT('',(-8.59702053001442E-15,2.45,-70.2));
#37937=CARTESIAN_POINT('',(-35.1,9.,60.7949833456676));
#37938=CARTESIAN_POINT('Origin',(1.55431223447522E-14,9.,2.22044604925031E-15));
#37939=CARTESIAN_POINT('',(-35.1,7.,60.7949833456676));
#37940=CARTESIAN_POINT('',(-35.1,5.,60.7949833456676));
#37941=CARTESIAN_POINT('',(-33.353701286408,5.,61.770305248534));
#37942=CARTESIAN_POINT('Ctrl Pts',(-35.1,7.,60.7949833456676));
#37943=CARTESIAN_POINT('Ctrl Pts',(-35.1,6.74887417302153,60.7949833456676));
#37944=CARTESIAN_POINT('Ctrl Pts',(-35.0565641212333,6.48100990452462,60.8201260037975));
#37945=CARTESIAN_POINT('Ctrl Pts',(-34.8795797765736,5.98825083345615,60.9217968358934));
#37946=CARTESIAN_POINT('Ctrl Pts',(-34.7459927648389,5.76335612152486,60.9982583355795));
#37947=CARTESIAN_POINT('Ctrl Pts',(-34.4369258181726,5.40818751436047,61.1732758953421));
#37948=CARTESIAN_POINT('Ctrl Pts',(-34.2408331115211,5.25425928439315,61.2834894043871));
#37949=CARTESIAN_POINT('Ctrl Pts',(-33.8097426473724,5.05016619199587,61.5223701418215));
#37950=CARTESIAN_POINT('Ctrl Pts',(-33.574708028271,5.,61.6509697066304));
#37951=CARTESIAN_POINT('Ctrl Pts',(-33.353701286408,5.,61.770305248534));
#37952=CARTESIAN_POINT('',(33.3537012864079,5.,61.770305248534));
#37953=CARTESIAN_POINT('Origin',(0.,5.,0.));
#37954=CARTESIAN_POINT('',(35.1,7.,60.7949833456676));
#37955=CARTESIAN_POINT('Ctrl Pts',(33.353701286408,5.,61.770305248534));
#37956=CARTESIAN_POINT('Ctrl Pts',(33.574708028271,5.,61.6509697066305));
#37957=CARTESIAN_POINT('Ctrl Pts',(33.8097426473723,5.05016619199587,61.5223701418215));
#37958=CARTESIAN_POINT('Ctrl Pts',(34.2408331115211,5.25425928439315,61.2834894043871));
#37959=CARTESIAN_POINT('Ctrl Pts',(34.4369258181726,5.40818751436047,61.1732758953421));
#37960=CARTESIAN_POINT('Ctrl Pts',(34.7459927648389,5.76335612152486,60.9982583355795));
#37961=CARTESIAN_POINT('Ctrl Pts',(34.8795797765736,5.98825083345615,60.9217968358934));
#37962=CARTESIAN_POINT('Ctrl Pts',(35.0565641212333,6.48100990452463,60.8201260037975));
#37963=CARTESIAN_POINT('Ctrl Pts',(35.1,6.74887417302153,60.7949833456676));
#37964=CARTESIAN_POINT('Ctrl Pts',(35.1,7.,60.7949833456676));
#37965=CARTESIAN_POINT('',(35.1,9.,60.7949833456676));
#37966=CARTESIAN_POINT('',(35.1,5.,60.7949833456676));
#37967=CARTESIAN_POINT('Origin',(1.55431223447522E-14,9.,2.22044604925031E-15));
#37968=CARTESIAN_POINT('Origin',(0.,7.,0.));
#37969=CARTESIAN_POINT('',(-2.70034619211991E-15,5.,-22.05));
#37970=CARTESIAN_POINT('Origin',(0.,5.,0.));
#37971=CARTESIAN_POINT('',(-2.45541683229044E-15,7.,-20.05));
#37972=CARTESIAN_POINT('Origin',(-2.70034619211991E-15,7.,-22.05));
#37973=CARTESIAN_POINT('Origin',(0.,7.,0.));
#37974=CARTESIAN_POINT('Origin',(0.,5.,20.05));
#37975=CARTESIAN_POINT('',(25.7497613597537,5.,48.5998949578673));
#37976=CARTESIAN_POINT('',(16.8589015289006,5.,33.2004740078565));
#37977=CARTESIAN_POINT('',(-25.7497613597537,5.,48.5998949578673));
#37978=CARTESIAN_POINT('',(-20.1589015289006,5.,38.9162416728338));
#37979=CARTESIAN_POINT('Origin',(-2.22044604925031E-15,5.,-1.11022302462516E-15));
#37980=CARTESIAN_POINT('Origin',(0.,17.5,0.));
#37981=CARTESIAN_POINT('',(-2.45541683229044E-15,30.,-20.05));
#37982=CARTESIAN_POINT('',(-2.45541683229044E-15,17.5,-20.05));
#37983=CARTESIAN_POINT('Origin',(0.,30.,0.));
#37984=CARTESIAN_POINT('Origin',(16.8589015289006,7.,33.2004740078565));
#37985=CARTESIAN_POINT('',(28.5,7.,49.363448015713));
#37986=CARTESIAN_POINT('',(18.5909523364695,7.,32.2004740078565));
#37987=CARTESIAN_POINT('Ctrl Pts',(25.7497613597537,5.,48.5998949578673));
#37988=CARTESIAN_POINT('Ctrl Pts',(25.7526780842804,5.,48.6007336279338));
#37989=CARTESIAN_POINT('Ctrl Pts',(25.7555948357263,5.00000332839376,48.6015722116644));
#37990=CARTESIAN_POINT('Ctrl Pts',(26.0511801116044,5.00067799125553,48.6865452392508));
#37991=CARTESIAN_POINT('Ctrl Pts',(26.3460171339481,5.03486692594129,48.7703312615877));
#37992=CARTESIAN_POINT('Ctrl Pts',(26.9009050741236,5.17036553160275,48.9263173337706));
#37993=CARTESIAN_POINT('Ctrl Pts',(27.1656717084766,5.26888612938734,48.9999335178016));
#37994=CARTESIAN_POINT('Ctrl Pts',(27.6543280663132,5.53732121577603,49.1345826791917));
#37995=CARTESIAN_POINT('Ctrl Pts',(27.8815247792677,5.70887974191627,49.1965246803542));
#37996=CARTESIAN_POINT('Ctrl Pts',(28.2058967874217,6.07814435711566,49.2844121204924));
#37997=CARTESIAN_POINT('Ctrl Pts',(28.3204632986599,6.25786799621181,49.3152504654719));
#37998=CARTESIAN_POINT('Ctrl Pts',(28.464178087957,6.63005485401211,49.3538606820259));
#37999=CARTESIAN_POINT('Ctrl Pts',(28.5,6.812926309153,49.363448015713));
#38000=CARTESIAN_POINT('Ctrl Pts',(28.5,7.,49.363448015713));
#38001=CARTESIAN_POINT('Origin',(-2.22044604925031E-15,7.,-1.11022302462516E-15));
#38002=CARTESIAN_POINT('',(-28.5,7.,49.363448015713));
#38003=CARTESIAN_POINT('Origin',(-2.22044604925031E-15,7.,-1.11022302462516E-15));
#38004=CARTESIAN_POINT('Ctrl Pts',(-25.7497613597537,5.,48.5998949578673));
#38005=CARTESIAN_POINT('Ctrl Pts',(-25.7526780842808,5.,48.6007336279339));
#38006=CARTESIAN_POINT('Ctrl Pts',(-25.7555948357259,5.00000332839376,48.6015722116643));
#38007=CARTESIAN_POINT('Ctrl Pts',(-26.0511801116162,5.00067799125556,48.6865452392533));
#38008=CARTESIAN_POINT('Ctrl Pts',(-26.34601713395,5.03486692594175,48.7703312615882));
#38009=CARTESIAN_POINT('Ctrl Pts',(-26.9009050741237,5.17036553160276,48.9263173337706));
#38010=CARTESIAN_POINT('Ctrl Pts',(-27.1656717084766,5.26888612938735,48.9999335178016));
#38011=CARTESIAN_POINT('Ctrl Pts',(-27.6543280663132,5.53732121577604,49.1345826791917));
#38012=CARTESIAN_POINT('Ctrl Pts',(-27.8815247792676,5.70887974191628,49.1965246803542));
#38013=CARTESIAN_POINT('Ctrl Pts',(-28.2058967874216,6.07814435711566,49.2844121204924));
#38014=CARTESIAN_POINT('Ctrl Pts',(-28.3204632986599,6.25786799621181,49.3152504654719));
#38015=CARTESIAN_POINT('Ctrl Pts',(-28.4641780879569,6.63005485401195,49.3538606820259));
#38016=CARTESIAN_POINT('Ctrl Pts',(-28.5,6.81292630915292,49.363448015713));
#38017=CARTESIAN_POINT('Ctrl Pts',(-28.5,7.,49.363448015713));
#38018=CARTESIAN_POINT('Origin',(-20.1589015289006,7.,38.9162416728338));
#38019=CARTESIAN_POINT('',(-21.8909523364695,7.,37.9162416728338));
#38020=CARTESIAN_POINT('Origin',(28.5,5.,49.363448015713));
#38021=CARTESIAN_POINT('',(28.5,9.,49.363448015713));
#38022=CARTESIAN_POINT('',(28.5,5.,49.363448015713));
#38023=CARTESIAN_POINT('',(35.1,9.,60.7949833456676));
#38024=CARTESIAN_POINT('Origin',(-2.22044604925031E-15,5.,-1.11022302462516E-15));
#38025=CARTESIAN_POINT('',(-28.5,9.,49.363448015713));
#38026=CARTESIAN_POINT('',(-28.5,5.,49.363448015713));
#38027=CARTESIAN_POINT('Origin',(-2.22044604925031E-15,9.,-1.11022302462516E-15));
#38028=CARTESIAN_POINT('Origin',(-35.1,5.,60.7949833456676));
#38029=CARTESIAN_POINT('',(-35.1,9.,60.7949833456676));
#38030=CARTESIAN_POINT('Origin',(90.,24.5,80.));
#38031=CARTESIAN_POINT('',(92.,8.,88.9057565652784));
#38032=CARTESIAN_POINT('',(90.,9.76000000000001,87.9558091983154));
#38033=CARTESIAN_POINT('Origin',(90.,8.,88.9057565652784));
#38034=CARTESIAN_POINT('',(90.0000000000017,24.5,96.75));
#38035=CARTESIAN_POINT('Origin',(90.,24.5,80.));
#38036=CARTESIAN_POINT('',(90.,39.24,87.9558091983154));
#38037=CARTESIAN_POINT('Origin',(90.,24.5,80.));
#38038=CARTESIAN_POINT('',(92.,41.,88.9057565652784));
#38039=CARTESIAN_POINT('Origin',(90.,41.,88.9057565652784));
#38040=CARTESIAN_POINT('Origin',(92.,24.5,80.));
#38041=CARTESIAN_POINT('Ctrl Pts',(90.,39.24,87.9558091983154));
#38042=CARTESIAN_POINT('Ctrl Pts',(90.,39.9925784091656,86.5614814216451));
#38043=CARTESIAN_POINT('Ctrl Pts',(89.6247663405678,40.8156274544267,84.3254689358931));
#38044=CARTESIAN_POINT('Ctrl Pts',(89.2998530158654,41.2636159206073,81.1945680459964));
#38045=CARTESIAN_POINT('Ctrl Pts',(89.2947826313174,41.2634913601257,78.0106147164496));
#38046=CARTESIAN_POINT('Ctrl Pts',(89.7999750759969,40.5929907863474,74.9075303285633));
#38047=CARTESIAN_POINT('Ctrl Pts',(90.0000000000018,39.6162892045687,72.7413546899905));
#38048=CARTESIAN_POINT('Ctrl Pts',(90.,39.2399999999846,72.0441908016561));
#38049=CARTESIAN_POINT('Ctrl Pts',(90.2991993003419,39.24,87.9558091983154));
#38050=CARTESIAN_POINT('Ctrl Pts',(90.3346190349092,40.0066898073963,86.535095061671));
#38051=CARTESIAN_POINT('Ctrl Pts',(90.0027743158155,40.8288120390463,84.2710725121084));
#38052=CARTESIAN_POINT('Ctrl Pts',(89.7146057062673,41.2627924802528,81.1713647613915));
#38053=CARTESIAN_POINT('Ctrl Pts',(89.7085874510504,41.2631573502512,78.0501047601331));
#38054=CARTESIAN_POINT('Ctrl Pts',(90.1626027926756,40.6115887482596,74.958234183941));
#38055=CARTESIAN_POINT('Ctrl Pts',(90.3169091676267,39.6233449036839,72.754547869977));
#38056=CARTESIAN_POINT('Ctrl Pts',(90.2991993003412,39.2399999999843,72.0441908016555));
#38057=CARTESIAN_POINT('Ctrl Pts',(90.8959652150226,39.3605997833875,88.0209020657502));
#38058=CARTESIAN_POINT('Ctrl Pts',(91.0015487583438,40.1907311515419,86.5517823378691));
#38059=CARTESIAN_POINT('Ctrl Pts',(90.7545425049392,41.0725721868577,84.2251614932142));
#38060=CARTESIAN_POINT('Ctrl Pts',(90.53851955239,41.5271753896422,81.1450147849467));
#38061=CARTESIAN_POINT('Ctrl Pts',(90.5305887720896,41.5281747157396,78.0951094062104));
#38062=CARTESIAN_POINT('Ctrl Pts',(90.8842946702604,40.8429080328149,74.9903449798908));
#38063=CARTESIAN_POINT('Ctrl Pts',(90.9487569866831,39.7756654674493,72.7136577981596));
#38064=CARTESIAN_POINT('Ctrl Pts',(90.8959652150205,39.3605997833705,71.9790979342197));
#38065=CARTESIAN_POINT('Ctrl Pts',(91.7377033118041,39.9492389941977,88.3386158546141));
#38066=CARTESIAN_POINT('Ctrl Pts',(91.8947737455775,40.9811300899403,86.8108756400174));
#38067=CARTESIAN_POINT('Ctrl Pts',(91.6657296933035,42.1250155322977,84.3862284321629));
#38068=CARTESIAN_POINT('Ctrl Pts',(91.4529882670294,42.7487257343339,81.1860321244351));
#38069=CARTESIAN_POINT('Ctrl Pts',(91.4440144391454,42.74912106062,78.0267860385529));
#38070=CARTESIAN_POINT('Ctrl Pts',(91.796936898285,41.8127986994321,74.7955406094651));
#38071=CARTESIAN_POINT('Ctrl Pts',(91.8162385286899,40.4651845420497,72.4252542526523));
#38072=CARTESIAN_POINT('Ctrl Pts',(91.7377033118009,39.9492389941766,71.6613841453547));
#38073=CARTESIAN_POINT('Ctrl Pts',(92.,40.6050569235487,88.6925888746107));
#38074=CARTESIAN_POINT('Ctrl Pts',(92.0842395543339,41.8020668522328,87.1438713820414));
#38075=CARTESIAN_POINT('Ctrl Pts',(91.675367371483,43.1416553165464,84.6695040349086));
#38076=CARTESIAN_POINT('Ctrl Pts',(91.304905483517,43.8870217698157,81.2798053980333));
#38077=CARTESIAN_POINT('Ctrl Pts',(91.2970139150286,43.8867145802671,77.8695340412403));
#38078=CARTESIAN_POINT('Ctrl Pts',(91.881114233009,42.7711777978807,74.486873307736));
#38079=CARTESIAN_POINT('Ctrl Pts',(92.0421197771678,41.2035618878683,72.0817698716415));
#38080=CARTESIAN_POINT('Ctrl Pts',(91.9999999999983,40.6050569235242,71.3074111253576));
#38081=CARTESIAN_POINT('Ctrl Pts',(92.,41.,88.9057565652784));
#38082=CARTESIAN_POINT('Ctrl Pts',(92.,42.2636577765839,87.3449418899014));
#38083=CARTESIAN_POINT('Ctrl Pts',(91.4371495108518,43.6456431137762,84.8419428386863));
#38084=CARTESIAN_POINT('Ctrl Pts',(90.9497795237981,44.3978625532585,81.3372030365632));
#38085=CARTESIAN_POINT('Ctrl Pts',(90.9421739469762,44.397653403196,77.7730761751302));
#38086=CARTESIAN_POINT('Ctrl Pts',(91.6999626139954,43.2718128875236,74.2994742483918));
#38087=CARTESIAN_POINT('Ctrl Pts',(92.0000000000027,41.6318288882683,71.8746507723773));
#38088=CARTESIAN_POINT('Ctrl Pts',(92.,40.9999999999741,71.0942434346896));
#38089=CARTESIAN_POINT('',(90.,39.2399999999846,72.0441908016561));
#38090=CARTESIAN_POINT('',(92.,40.9999999999871,71.0942434346896));
#38091=CARTESIAN_POINT('Origin',(90.,40.9999999999828,71.0942434346896));
#38092=CARTESIAN_POINT('Ctrl Pts',(92.,40.9999999999741,71.0942434346896));
#38093=CARTESIAN_POINT('Ctrl Pts',(92.0000000000027,41.6318288882683,71.8746507723773));
#38094=CARTESIAN_POINT('Ctrl Pts',(91.6999626139954,43.2718128875236,74.2994742483918));
#38095=CARTESIAN_POINT('Ctrl Pts',(90.9421739469762,44.397653403196,77.7730761751302));
#38096=CARTESIAN_POINT('Ctrl Pts',(90.9497795237981,44.3978625532585,81.3372030365632));
#38097=CARTESIAN_POINT('Ctrl Pts',(91.4371495108518,43.6456431137762,84.8419428386863));
#38098=CARTESIAN_POINT('Ctrl Pts',(92.,42.2636577765839,87.3449418899014));
#38099=CARTESIAN_POINT('Ctrl Pts',(92.,41.,88.9057565652784));
#38100=CARTESIAN_POINT('Ctrl Pts',(90.,39.24,87.9558091983154));
#38101=CARTESIAN_POINT('Ctrl Pts',(90.,39.9925784091656,86.5614814216451));
#38102=CARTESIAN_POINT('Ctrl Pts',(89.6247663405678,40.8156274544267,84.3254689358931));
#38103=CARTESIAN_POINT('Ctrl Pts',(89.2998530158654,41.2636159206073,81.1945680459964));
#38104=CARTESIAN_POINT('Ctrl Pts',(89.2947826313174,41.2634913601257,78.0106147164496));
#38105=CARTESIAN_POINT('Ctrl Pts',(89.7999750759969,40.5929907863474,74.9075303285633));
#38106=CARTESIAN_POINT('Ctrl Pts',(90.0000000000018,39.6162892045687,72.7413546899905));
#38107=CARTESIAN_POINT('Ctrl Pts',(90.,39.2399999999846,72.0441908016561));
#38108=CARTESIAN_POINT('Origin',(90.,24.5,80.));
#38109=CARTESIAN_POINT('',(90.,9.76,72.0441908016846));
#38110=CARTESIAN_POINT('',(92.,8.,71.0942434347216));
#38111=CARTESIAN_POINT('Origin',(90.,8.,71.0942434347216));
#38112=CARTESIAN_POINT('Origin',(92.,24.5,80.));
#38113=CARTESIAN_POINT('Origin',(90.,24.5,80.));
#38114=CARTESIAN_POINT('Ctrl Pts',(90.,9.75999999999999,72.0441908016846));
#38115=CARTESIAN_POINT('Ctrl Pts',(90.,9.0074215908359,73.4385185783522));
#38116=CARTESIAN_POINT('Ctrl Pts',(89.6266311441226,8.1845886271713,75.6741761987655));
#38117=CARTESIAN_POINT('Ctrl Pts',(89.2991132263711,7.73666063782126,78.8058465499708));
#38118=CARTESIAN_POINT('Ctrl Pts',(89.3000459409121,7.73672873935593,81.19334048201));
#38119=CARTESIAN_POINT('Ctrl Pts',(89.6267478600051,8.18449985726607,84.325124610408));
#38120=CARTESIAN_POINT('Ctrl Pts',(90.,9.00742159083591,86.5614814216478));
#38121=CARTESIAN_POINT('Ctrl Pts',(90.,9.76,87.9558091983154));
#38122=CARTESIAN_POINT('Ctrl Pts',(90.2991993003419,9.75999999999999,72.0441908016846));
#38123=CARTESIAN_POINT('Ctrl Pts',(90.3346190349092,8.99331019260512,73.4649049383263));
#38124=CARTESIAN_POINT('Ctrl Pts',(90.0050584632404,8.1716440685805,75.728826404617));
#38125=CARTESIAN_POINT('Ctrl Pts',(89.7138584041868,7.7375255864327,78.8287976868203));
#38126=CARTESIAN_POINT('Ctrl Pts',(89.7146849504547,7.73748906209263,81.1706049698146));
#38127=CARTESIAN_POINT('Ctrl Pts',(90.0052338960302,8.17159823794263,84.2702498335073));
#38128=CARTESIAN_POINT('Ctrl Pts',(90.3346190349092,8.99331019260513,86.5350950616738));
#38129=CARTESIAN_POINT('Ctrl Pts',(90.2991993003419,9.76,87.9558091983154));
#38130=CARTESIAN_POINT('Ctrl Pts',(90.895972204776,9.639403332612,71.9790996160882));
#38131=CARTESIAN_POINT('Ctrl Pts',(91.001555748097,8.80927196445914,73.4482193439664));
#38132=CARTESIAN_POINT('Ctrl Pts',(90.7577009802419,7.92816993286539,75.7750896491985));
#38133=CARTESIAN_POINT('Ctrl Pts',(90.5378845432001,7.47299912767311,78.8547095061753));
#38134=CARTESIAN_POINT('Ctrl Pts',(90.5384579232711,7.47292007731554,81.1450808709336));
#38135=CARTESIAN_POINT('Ctrl Pts',(90.7580323548137,7.92805069968786,84.2236005862538));
#38136=CARTESIAN_POINT('Ctrl Pts',(91.001555748097,8.80927196445915,86.5517806560335));
#38137=CARTESIAN_POINT('Ctrl Pts',(90.895972204776,9.639403332612,88.0209003839118));
#38138=CARTESIAN_POINT('Ctrl Pts',(91.7377173103273,9.05076546339944,71.661386551342));
#38139=CARTESIAN_POINT('Ctrl Pts',(91.8947877441005,8.01887436765872,73.189126765936));
#38140=CARTESIAN_POINT('Ctrl Pts',(91.6692926181241,6.87547810564428,75.614027382202));
#38141=CARTESIAN_POINT('Ctrl Pts',(91.4520070536192,6.25140468377173,78.8135720334519));
#38142=CARTESIAN_POINT('Ctrl Pts',(91.452718603279,6.25149630787978,81.1863103961658));
#38143=CARTESIAN_POINT('Ctrl Pts',(91.6695544894331,6.87512702275017,84.3845380263156));
#38144=CARTESIAN_POINT('Ctrl Pts',(91.8947877441005,8.01887436765873,86.810873234064));
#38145=CARTESIAN_POINT('Ctrl Pts',(91.7377173103273,9.05076546339944,88.338613448658));
#38146=CARTESIAN_POINT('Ctrl Pts',(92.,8.39494307645129,71.3074111253893));
#38147=CARTESIAN_POINT('Ctrl Pts',(92.0842395543337,7.19793314776939,72.8561286179559));
#38148=CARTESIAN_POINT('Ctrl Pts',(91.678416051393,5.8585488221207,75.3303789281826));
#38149=CARTESIAN_POINT('Ctrl Pts',(91.304319836793,5.11301911897351,78.7203674934503));
#38150=CARTESIAN_POINT('Ctrl Pts',(91.3052869701975,5.11331092315558,81.2790379801232));
#38151=CARTESIAN_POINT('Ctrl Pts',(91.6787682642829,5.85813477479916,84.6685518615818));
#38152=CARTESIAN_POINT('Ctrl Pts',(92.0842395543337,7.1979331477694,87.1438713820441));
#38153=CARTESIAN_POINT('Ctrl Pts',(92.,8.39494307645129,88.6925888746107));
#38154=CARTESIAN_POINT('Ctrl Pts',(92.,8.00000000000001,71.0942434347216));
#38155=CARTESIAN_POINT('Ctrl Pts',(92.,6.73634222341846,72.6550581100958));
#38156=CARTESIAN_POINT('Ctrl Pts',(91.4399467161839,5.35471970980254,75.1576599239912));
#38157=CARTESIAN_POINT('Ctrl Pts',(90.9486698395567,4.60260181723717,78.6632610634002));
#38158=CARTESIAN_POINT('Ctrl Pts',(90.9500689113682,4.60271616682896,81.3358288977724));
#38159=CARTESIAN_POINT('Ctrl Pts',(91.4401217900076,5.35457065585718,84.8415573997105));
#38160=CARTESIAN_POINT('Ctrl Pts',(92.,6.73634222341846,87.3449418899042));
#38161=CARTESIAN_POINT('Ctrl Pts',(92.,8.00000000000001,88.9057565652784));
#38162=CARTESIAN_POINT('Ctrl Pts',(92.,8.00000000000001,88.9057565652784));
#38163=CARTESIAN_POINT('Ctrl Pts',(92.,6.73634222341846,87.3449418899042));
#38164=CARTESIAN_POINT('Ctrl Pts',(91.4401217900076,5.35457065585718,84.8415573997105));
#38165=CARTESIAN_POINT('Ctrl Pts',(90.9500689113682,4.60271616682896,81.3358288977724));
#38166=CARTESIAN_POINT('Ctrl Pts',(90.9486698395567,4.60260181723717,78.6632610634002));
#38167=CARTESIAN_POINT('Ctrl Pts',(91.4399467161839,5.35471970980254,75.1576599239912));
#38168=CARTESIAN_POINT('Ctrl Pts',(92.,6.73634222341846,72.6550581100958));
#38169=CARTESIAN_POINT('Ctrl Pts',(92.,8.00000000000001,71.0942434347216));
#38170=CARTESIAN_POINT('Ctrl Pts',(90.,9.75999999999999,72.0441908016846));
#38171=CARTESIAN_POINT('Ctrl Pts',(90.,9.0074215908359,73.4385185783522));
#38172=CARTESIAN_POINT('Ctrl Pts',(89.6266311441226,8.1845886271713,75.6741761987655));
#38173=CARTESIAN_POINT('Ctrl Pts',(89.2991132263711,7.73666063782126,78.8058465499708));
#38174=CARTESIAN_POINT('Ctrl Pts',(89.3000459409121,7.73672873935593,81.19334048201));
#38175=CARTESIAN_POINT('Ctrl Pts',(89.6267478600051,8.18449985726607,84.325124610408));
#38176=CARTESIAN_POINT('Ctrl Pts',(90.,9.00742159083591,86.5614814216478));
#38177=CARTESIAN_POINT('Ctrl Pts',(90.,9.76,87.9558091983154));
#38178=CARTESIAN_POINT('Origin',(86.,7.99999999999997,50.));
#38179=CARTESIAN_POINT('',(92.,8.,108.));
#38180=CARTESIAN_POINT('',(92.,8.,50.));
#38181=CARTESIAN_POINT('',(86.,2.,108.));
#38182=CARTESIAN_POINT('Origin',(86.,7.99999999999997,108.));
#38183=CARTESIAN_POINT('',(86.,2.,50.));
#38184=CARTESIAN_POINT('',(86.,2.,50.));
#38185=CARTESIAN_POINT('',(92.,8.,50.));
#38186=CARTESIAN_POINT('Origin',(86.,7.99999999999997,50.));
#38187=CARTESIAN_POINT('',(92.,8.,50.));
#38188=CARTESIAN_POINT('Origin',(92.,8.,50.));
#38189=CARTESIAN_POINT('',(92.,41.,108.));
#38190=CARTESIAN_POINT('',(92.,41.,50.));
#38191=CARTESIAN_POINT('',(92.,16.25,108.));
#38192=CARTESIAN_POINT('Origin',(92.,24.5,80.));
#38193=CARTESIAN_POINT('',(70.,24.5,96.75));
#38194=CARTESIAN_POINT('',(92.,24.5,96.75));
#38195=CARTESIAN_POINT('Origin',(70.,24.5,80.));
#38196=CARTESIAN_POINT('Origin',(43.,45.,52.));
#38197=CARTESIAN_POINT('',(-86.,45.,50.));
#38198=CARTESIAN_POINT('',(43.,45.,50.));
#38199=CARTESIAN_POINT('',(-86.,47.,52.));
#38200=CARTESIAN_POINT('Origin',(-86.,45.,52.));
#38201=CARTESIAN_POINT('',(43.,47.,52.));
#38202=CARTESIAN_POINT('Origin',(-90.,32.75,52.));
#38203=CARTESIAN_POINT('',(-92.,41.,52.));
#38204=CARTESIAN_POINT('',(-90.,41.,50.));
#38205=CARTESIAN_POINT('Origin',(-90.,41.,52.));
#38206=CARTESIAN_POINT('',(-90.,8.,50.));
#38207=CARTESIAN_POINT('',(-90.,32.75,50.));
#38208=CARTESIAN_POINT('',(-92.,8.,52.));
#38209=CARTESIAN_POINT('Origin',(-90.,8.,52.));
#38210=CARTESIAN_POINT('',(-92.,32.75,52.));
#38211=CARTESIAN_POINT('Origin',(-86.,7.99999999999997,52.));
#38212=CARTESIAN_POINT('',(-86.,4.00000000000001,50.));
#38213=CARTESIAN_POINT('',(-86.,2.00000000000001,52.));
#38214=CARTESIAN_POINT('Origin',(-86.,4.00000000000001,52.));
#38215=CARTESIAN_POINT('Origin',(-86.,7.99999999999997,52.));
#38216=CARTESIAN_POINT('Origin',(-86.,7.99999999999997,50.));
#38217=CARTESIAN_POINT('Origin',(-43.,4.,52.));
#38218=CARTESIAN_POINT('',(-43.,2.,52.));
#38219=CARTESIAN_POINT('',(-43.,4.,50.));
#38220=CARTESIAN_POINT('Origin',(-86.,41.,52.));
#38221=CARTESIAN_POINT('Origin',(-86.,41.,52.));
#38222=CARTESIAN_POINT('Origin',(-86.,41.,50.));
#38223=CARTESIAN_POINT('Origin',(-86.,7.99999999999997,50.));
#38224=CARTESIAN_POINT('',(-86.,2.00000000000001,108.));
#38225=CARTESIAN_POINT('',(-86.,2.00000000000001,50.));
#38226=CARTESIAN_POINT('',(-92.,8.,108.));
#38227=CARTESIAN_POINT('Origin',(-86.,7.99999999999997,108.));
#38228=CARTESIAN_POINT('',(-92.,8.,88.9057565652784));
#38229=CARTESIAN_POINT('',(-92.,8.,50.));
#38230=CARTESIAN_POINT('',(-92.,8.00000000001294,71.0942434346896));
#38231=CARTESIAN_POINT('Ctrl Pts',(-92.,8.00000000002587,71.0942434346896));
#38232=CARTESIAN_POINT('Ctrl Pts',(-92.0000000000041,7.05225666758454,72.2648544412212));
#38233=CARTESIAN_POINT('Ctrl Pts',(-91.713227279185,6.04343085354599,73.9095997432177));
#38234=CARTESIAN_POINT('Ctrl Pts',(-91.255731456336,5.07242771945905,76.4722824902359));
#38235=CARTESIAN_POINT('Ctrl Pts',(-90.947934136765,4.60143957017688,78.6641302175159));
#38236=CARTESIAN_POINT('Ctrl Pts',(-90.942940568041,4.6025640632853,82.2271784882658));
#38237=CARTESIAN_POINT('Ctrl Pts',(-91.6991668412039,5.72806963647306,85.7013212348271));
#38238=CARTESIAN_POINT('Ctrl Pts',(-92.,7.36817111170808,88.1253492275899));
#38239=CARTESIAN_POINT('Ctrl Pts',(-92.,8.00000000000001,88.9057565652784));
#38240=CARTESIAN_POINT('',(-92.,8.,50.));
#38241=CARTESIAN_POINT('Origin',(-86.,2.,50.));
#38242=CARTESIAN_POINT('',(-86.,2.,50.));
#38243=CARTESIAN_POINT('',(-43.,2.,108.));
#38244=CARTESIAN_POINT('Origin',(0.,24.5,50.));
#38245=CARTESIAN_POINT('Origin',(-90.,32.75,108.));
#38246=CARTESIAN_POINT('',(-90.,41.,110.));
#38247=CARTESIAN_POINT('',(-92.,41.,108.));
#38248=CARTESIAN_POINT('Origin',(-90.,41.,108.));
#38249=CARTESIAN_POINT('',(-92.,32.75,108.));
#38250=CARTESIAN_POINT('',(-90.,8.,110.));
#38251=CARTESIAN_POINT('Origin',(-90.,8.,108.));
#38252=CARTESIAN_POINT('',(-90.,32.75,110.));
#38253=CARTESIAN_POINT('Origin',(-86.,7.99999999999997,108.));
#38254=CARTESIAN_POINT('',(-86.,4.00000000000001,110.));
#38255=CARTESIAN_POINT('Origin',(-86.,4.00000000000001,108.));
#38256=CARTESIAN_POINT('Origin',(-86.,7.99999999999997,110.));
#38257=CARTESIAN_POINT('Origin',(-43.,4.,108.));
#38258=CARTESIAN_POINT('',(86.,4.,110.));
#38259=CARTESIAN_POINT('Origin',(86.,4.,108.));
#38260=CARTESIAN_POINT('',(-43.,4.,110.));
#38261=CARTESIAN_POINT('Origin',(86.,7.99999999999997,108.));
#38262=CARTESIAN_POINT('',(90.,7.99999999999999,110.));
#38263=CARTESIAN_POINT('Origin',(90.,7.99999999999999,108.));
#38264=CARTESIAN_POINT('Origin',(86.,7.99999999999997,110.));
#38265=CARTESIAN_POINT('Origin',(90.,16.25,108.));
#38266=CARTESIAN_POINT('',(90.,41.,110.));
#38267=CARTESIAN_POINT('Origin',(90.,41.,108.));
#38268=CARTESIAN_POINT('',(90.,16.25,110.));
#38269=CARTESIAN_POINT('Origin',(86.,41.,108.));
#38270=CARTESIAN_POINT('',(86.,47.,108.));
#38271=CARTESIAN_POINT('',(86.,45.,110.));
#38272=CARTESIAN_POINT('Origin',(86.,45.,108.));
#38273=CARTESIAN_POINT('Origin',(86.,41.,110.));
#38274=CARTESIAN_POINT('Origin',(86.,41.,108.));
#38275=CARTESIAN_POINT('Origin',(43.,45.,108.));
#38276=CARTESIAN_POINT('',(-86.,47.,108.));
#38277=CARTESIAN_POINT('',(-86.,45.,110.));
#38278=CARTESIAN_POINT('Origin',(-86.,45.,108.));
#38279=CARTESIAN_POINT('',(43.,45.,110.));
#38280=CARTESIAN_POINT('',(43.,47.,108.));
#38281=CARTESIAN_POINT('Origin',(-86.,41.,108.));
#38282=CARTESIAN_POINT('Origin',(-86.,41.,110.));
#38283=CARTESIAN_POINT('Origin',(-86.,41.,108.));
#38284=CARTESIAN_POINT('Origin',(-92.,41.,50.));
#38285=CARTESIAN_POINT('',(-92.,41.,88.9057565652784));
#38286=CARTESIAN_POINT('',(-92.,41.,50.));
#38287=CARTESIAN_POINT('Origin',(-92.,24.5,80.));
#38288=CARTESIAN_POINT('Origin',(0.,24.5,110.));
#38289=CARTESIAN_POINT('',(-51.,33.5,110.));
#38290=CARTESIAN_POINT('Origin',(-51.,30.5,110.));
#38291=CARTESIAN_POINT('',(-39.,33.5,110.));
#38292=CARTESIAN_POINT('',(-19.5,33.5,110.));
#38293=CARTESIAN_POINT('',(-36.,30.5,110.));
#38294=CARTESIAN_POINT('Origin',(-39.,30.5,110.));
#38295=CARTESIAN_POINT('',(-36.,21.5,110.));
#38296=CARTESIAN_POINT('',(39.,33.5,110.));
#38297=CARTESIAN_POINT('Origin',(39.,30.5,110.));
#38298=CARTESIAN_POINT('',(51.,33.5,110.));
#38299=CARTESIAN_POINT('',(25.5,33.5,110.));
#38300=CARTESIAN_POINT('',(54.,30.5,110.));
#38301=CARTESIAN_POINT('Origin',(51.,30.5,110.));
#38302=CARTESIAN_POINT('',(54.,21.5,110.));
#38303=CARTESIAN_POINT('',(-16.75,24.5,110.));
#38304=CARTESIAN_POINT('Origin',(0.,24.5,110.));
#38305=CARTESIAN_POINT('Origin',(-90.,24.5,80.));
#38306=CARTESIAN_POINT('',(-90.,39.24,87.9558091983154));
#38307=CARTESIAN_POINT('Origin',(-90.,41.,88.9057565652784));
#38308=CARTESIAN_POINT('',(-90.0000000000017,24.5,96.75));
#38309=CARTESIAN_POINT('Origin',(-90.,24.5,80.));
#38310=CARTESIAN_POINT('',(-90.,9.76000000000001,87.9558091983154));
#38311=CARTESIAN_POINT('Origin',(-90.,24.5,80.));
#38312=CARTESIAN_POINT('Origin',(-90.,8.,88.9057565652784));
#38313=CARTESIAN_POINT('Ctrl Pts',(-90.,9.76,87.9558091983154));
#38314=CARTESIAN_POINT('Ctrl Pts',(-90.,9.38371079541722,87.2586453099802));
#38315=CARTESIAN_POINT('Ctrl Pts',(-89.7994445608026,8.40693925016618,85.0931803031121));
#38316=CARTESIAN_POINT('Ctrl Pts',(-89.2952937120273,7.73663815324546,81.9896127828507));
#38317=CARTESIAN_POINT('Ctrl Pts',(-89.2986227578434,7.73596845512756,78.8066229943142));
#38318=CARTESIAN_POINT('Ctrl Pts',(-89.5038209708906,8.01646806403338,76.8485723579441));
#38319=CARTESIAN_POINT('Ctrl Pts',(-89.8088181861233,8.59475437500072,74.5592424372745));
#38320=CARTESIAN_POINT('Ctrl Pts',(-90.0000000000027,9.19556619313921,73.0899366341577));
#38321=CARTESIAN_POINT('Ctrl Pts',(-90.,9.7600000000154,72.0441908016561));
#38322=CARTESIAN_POINT('Ctrl Pts',(-90.2991993003419,9.76,87.9558091983154));
#38323=CARTESIAN_POINT('Ctrl Pts',(-90.3169091676255,9.37665509630183,87.2454521299932));
#38324=CARTESIAN_POINT('Ctrl Pts',(-90.1619476924458,8.38826138246784,85.0425306128612));
#38325=CARTESIAN_POINT('Ctrl Pts',(-89.7091767454643,7.73701774875792,81.9500740924077));
#38326=CARTESIAN_POINT('Ctrl Pts',(-89.7131477349571,7.73663955285474,78.8298975124876));
#38327=CARTESIAN_POINT('Ctrl Pts',(-89.8958101886172,8.00865749204959,76.8911873219261));
#38328=CARTESIAN_POINT('Ctrl Pts',(-90.1644704238476,8.58067298580855,74.599875320748));
#38329=CARTESIAN_POINT('Ctrl Pts',(-90.3257641012695,9.18498264446627,73.1097264041378));
#38330=CARTESIAN_POINT('Ctrl Pts',(-90.2991993003412,9.76000000001569,72.0441908016555));
#38331=CARTESIAN_POINT('Ctrl Pts',(-90.895972204776,9.63940333261201,88.0209003839118));
#38332=CARTESIAN_POINT('Ctrl Pts',(-90.9487639764366,9.2243376485348,87.2863405199713));
#38333=CARTESIAN_POINT('Ctrl Pts',(-90.8833386248301,8.15696353645985,85.0104469472155));
#38334=CARTESIAN_POINT('Ctrl Pts',(-90.5313266508363,7.47206531180379,81.9050471896105));
#38335=CARTESIAN_POINT('Ctrl Pts',(-90.5365149718603,7.47226163348177,78.8562489519795));
#38336=CARTESIAN_POINT('Ctrl Pts',(-90.6750800382882,7.75723042413783,76.9297385435099));
#38337=CARTESIAN_POINT('Ctrl Pts',(-90.8723012998031,8.36666124302361,74.6145362955887));
#38338=CARTESIAN_POINT('Ctrl Pts',(-90.9751598622677,9.01680480651077,73.080939411968));
#38339=CARTESIAN_POINT('Ctrl Pts',(-90.8959722047739,9.63940333262899,71.9790996160581));
#38340=CARTESIAN_POINT('Ctrl Pts',(-91.7377173103273,9.05076546339945,88.338613448658));
#38341=CARTESIAN_POINT('Ctrl Pts',(-91.8162525272141,8.53481991552815,87.5747433413596));
#38342=CARTESIAN_POINT('Ctrl Pts',(-91.7960385570055,7.18720898037985,85.2052170002644));
#38343=CARTESIAN_POINT('Ctrl Pts',(-91.4449131702562,6.25099366023525,81.9734225373038));
#38344=CARTESIAN_POINT('Ctrl Pts',(-91.4510308374062,6.25092309230086,78.8151638422316));
#38345=CARTESIAN_POINT('Ctrl Pts',(-91.587647686046,6.64111672717885,76.813793060011));
#38346=CARTESIAN_POINT('Ctrl Pts',(-91.7743660572492,7.44592541337458,74.4042344174921));
#38347=CARTESIAN_POINT('Ctrl Pts',(-91.8555201356577,8.2768471416109,72.8071917122573));
#38348=CARTESIAN_POINT('Ctrl Pts',(-91.7377173103241,9.05076546342056,71.6613865513108));
#38349=CARTESIAN_POINT('Ctrl Pts',(-92.,8.3949430764513,88.6925888746107));
#38350=CARTESIAN_POINT('Ctrl Pts',(-92.0421197771669,7.79643811210926,87.9182301283261));
#38351=CARTESIAN_POINT('Ctrl Pts',(-91.8800131297229,6.2289539284548,85.5139158134625));
#38352=CARTESIAN_POINT('Ctrl Pts',(-91.297671044354,5.1134253012412,82.1307014026271));
#38353=CARTESIAN_POINT('Ctrl Pts',(-91.3026286831461,5.11277842806216,78.7214477499932));
#38354=CARTESIAN_POINT('Ctrl Pts',(-91.5379503533126,5.57872018718012,76.6015467847076));
#38355=CARTESIAN_POINT('Ctrl Pts',(-91.8735935522416,6.52745583762372,74.0962088888192));
#38356=CARTESIAN_POINT('Ctrl Pts',(-92.0631796657526,7.49718562995966,72.4689492447835));
#38357=CARTESIAN_POINT('Ctrl Pts',(-91.9999999999983,8.39494307647579,71.3074111253576));
#38358=CARTESIAN_POINT('Ctrl Pts',(-92.,8.00000000000001,88.9057565652784));
#38359=CARTESIAN_POINT('Ctrl Pts',(-92.,7.36817111170808,88.1253492275899));
#38360=CARTESIAN_POINT('Ctrl Pts',(-91.6991668412039,5.72806963647306,85.7013212348271));
#38361=CARTESIAN_POINT('Ctrl Pts',(-90.942940568041,4.6025640632853,82.2271784882658));
#38362=CARTESIAN_POINT('Ctrl Pts',(-90.947934136765,4.60143957017688,78.6641302175159));
#38363=CARTESIAN_POINT('Ctrl Pts',(-91.255731456336,5.07242771945905,76.4722824902359));
#38364=CARTESIAN_POINT('Ctrl Pts',(-91.713227279185,6.04343085354599,73.9095997432177));
#38365=CARTESIAN_POINT('Ctrl Pts',(-92.0000000000041,7.05225666758454,72.2648544412212));
#38366=CARTESIAN_POINT('Ctrl Pts',(-92.,8.00000000002587,71.0942434346896));
#38367=CARTESIAN_POINT('',(-90.,9.7600000000154,72.0441908016561));
#38368=CARTESIAN_POINT('Origin',(-90.,8.00000000001724,71.0942434346896));
#38369=CARTESIAN_POINT('Ctrl Pts',(-90.,9.76,87.9558091983154));
#38370=CARTESIAN_POINT('Ctrl Pts',(-90.,9.38371079541722,87.2586453099802));
#38371=CARTESIAN_POINT('Ctrl Pts',(-89.7994445608026,8.40693925016618,85.0931803031121));
#38372=CARTESIAN_POINT('Ctrl Pts',(-89.2952937120273,7.73663815324546,81.9896127828507));
#38373=CARTESIAN_POINT('Ctrl Pts',(-89.2986227578434,7.73596845512756,78.8066229943142));
#38374=CARTESIAN_POINT('Ctrl Pts',(-89.5038209708906,8.01646806403338,76.8485723579441));
#38375=CARTESIAN_POINT('Ctrl Pts',(-89.8088181861233,8.59475437500072,74.5592424372745));
#38376=CARTESIAN_POINT('Ctrl Pts',(-90.0000000000027,9.19556619313921,73.0899366341577));
#38377=CARTESIAN_POINT('Ctrl Pts',(-90.,9.7600000000154,72.0441908016561));
#38378=CARTESIAN_POINT('Origin',(-90.,24.5,80.));
#38379=CARTESIAN_POINT('',(-90.,39.24,72.0441908016846));
#38380=CARTESIAN_POINT('',(-92.,41.,71.0942434347216));
#38381=CARTESIAN_POINT('Origin',(-90.,41.,71.0942434347216));
#38382=CARTESIAN_POINT('Origin',(-92.,24.5,80.));
#38383=CARTESIAN_POINT('Origin',(-90.,24.5,80.));
#38384=CARTESIAN_POINT('Ctrl Pts',(-90.,39.24,72.0441908016846));
#38385=CARTESIAN_POINT('Ctrl Pts',(-90.,39.9925784091641,73.4385185783522));
#38386=CARTESIAN_POINT('Ctrl Pts',(-89.6247663405693,40.8156274544243,75.6745310640996));
#38387=CARTESIAN_POINT('Ctrl Pts',(-89.2998530158664,41.2636159206061,78.8054319539897));
#38388=CARTESIAN_POINT('Ctrl Pts',(-89.2947826313159,41.2634913601276,81.9893852835302));
#38389=CARTESIAN_POINT('Ctrl Pts',(-89.7999750759925,40.5929907863548,85.0924696714116));
#38390=CARTESIAN_POINT('Ctrl Pts',(-90.,39.616289204582,87.2586453099816));
#38391=CARTESIAN_POINT('Ctrl Pts',(-90.,39.24,87.9558091983154));
#38392=CARTESIAN_POINT('Ctrl Pts',(-90.2991993003419,39.24,72.0441908016846));
#38393=CARTESIAN_POINT('Ctrl Pts',(-90.3346190349092,40.0066898073949,73.4649049383262));
#38394=CARTESIAN_POINT('Ctrl Pts',(-90.0027743158169,40.8288120390438,75.7289274878841));
#38395=CARTESIAN_POINT('Ctrl Pts',(-89.7146057062682,41.2627924802516,78.8286352385948));
#38396=CARTESIAN_POINT('Ctrl Pts',(-89.7085874510491,41.263157350253,81.9498952398471));
#38397=CARTESIAN_POINT('Ctrl Pts',(-90.1626027926716,40.6115887482669,85.0417658160337));
#38398=CARTESIAN_POINT('Ctrl Pts',(-90.3169091676255,39.6233449036974,87.2454521299946));
#38399=CARTESIAN_POINT('Ctrl Pts',(-90.2991993003419,39.24,87.9558091983154));
#38400=CARTESIAN_POINT('Ctrl Pts',(-90.8959652150227,39.3605997833875,71.9790979342498));
#38401=CARTESIAN_POINT('Ctrl Pts',(-91.0015487583436,40.1907311515403,73.4482176621281));
#38402=CARTESIAN_POINT('Ctrl Pts',(-90.7545425049403,41.0725721868551,75.7748385067781));
#38403=CARTESIAN_POINT('Ctrl Pts',(-90.5385195523907,41.527175389641,78.8549852150399));
#38404=CARTESIAN_POINT('Ctrl Pts',(-90.5305887720886,41.5281747157414,81.9048905937702));
#38405=CARTESIAN_POINT('Ctrl Pts',(-90.8842946702573,40.8429080328227,85.0096550200834));
#38406=CARTESIAN_POINT('Ctrl Pts',(-90.9487569866832,39.7756654674639,87.2863422018111));
#38407=CARTESIAN_POINT('Ctrl Pts',(-90.8959652150227,39.3605997833875,88.0209020657502));
#38408=CARTESIAN_POINT('Ctrl Pts',(-91.7377033118041,39.9492389941977,71.6613841453859));
#38409=CARTESIAN_POINT('Ctrl Pts',(-91.8947737455773,40.9811300899385,73.1891243599799));
#38410=CARTESIAN_POINT('Ctrl Pts',(-91.6657296933045,42.1250155322943,75.6137715678291));
#38411=CARTESIAN_POINT('Ctrl Pts',(-91.45298826703,42.7487257343322,78.813967875551));
#38412=CARTESIAN_POINT('Ctrl Pts',(-91.4440144391444,42.7491210606227,81.9732139614271));
#38413=CARTESIAN_POINT('Ctrl Pts',(-91.796936898282,41.8127986994424,85.204459390508));
#38414=CARTESIAN_POINT('Ctrl Pts',(-91.8162385286907,40.465184542068,87.5747457473173));
#38415=CARTESIAN_POINT('Ctrl Pts',(-91.7377033118041,39.9492389941978,88.3386158546141));
#38416=CARTESIAN_POINT('Ctrl Pts',(-92.,40.6050569235487,71.3074111253893));
#38417=CARTESIAN_POINT('Ctrl Pts',(-92.0842395543337,41.8020668522306,72.8561286179559));
#38418=CARTESIAN_POINT('Ctrl Pts',(-91.6753673714846,43.1416553165424,75.3304959650833));
#38419=CARTESIAN_POINT('Ctrl Pts',(-91.3049054835182,43.8870217698137,78.7201946019518));
#38420=CARTESIAN_POINT('Ctrl Pts',(-91.2970139150267,43.8867145802703,82.1304659587381));
#38421=CARTESIAN_POINT('Ctrl Pts',(-91.8811142330039,42.7711777978929,85.5131266922364));
#38422=CARTESIAN_POINT('Ctrl Pts',(-92.0421197771668,41.2035618878896,87.9182301283276));
#38423=CARTESIAN_POINT('Ctrl Pts',(-92.,40.6050569235487,88.6925888746107));
#38424=CARTESIAN_POINT('Ctrl Pts',(-92.,41.,71.0942434347216));
#38425=CARTESIAN_POINT('Ctrl Pts',(-92.,42.2636577765815,72.6550581100958));
#38426=CARTESIAN_POINT('Ctrl Pts',(-91.4371495108539,43.6456431137721,75.1580571613055));
#38427=CARTESIAN_POINT('Ctrl Pts',(-90.9497795237996,44.3978625532565,78.6627969634214));
#38428=CARTESIAN_POINT('Ctrl Pts',(-90.9421739469738,44.3976534031992,82.2269238248473));
#38429=CARTESIAN_POINT('Ctrl Pts',(-91.6999626139887,43.271812887536,85.7005257515802));
#38430=CARTESIAN_POINT('Ctrl Pts',(-92.,41.6318288882907,88.1253492275915));
#38431=CARTESIAN_POINT('Ctrl Pts',(-92.,41.,88.9057565652784));
#38432=CARTESIAN_POINT('Ctrl Pts',(-92.,41.,88.9057565652784));
#38433=CARTESIAN_POINT('Ctrl Pts',(-92.,41.6318288882907,88.1253492275915));
#38434=CARTESIAN_POINT('Ctrl Pts',(-91.6999626139887,43.271812887536,85.7005257515802));
#38435=CARTESIAN_POINT('Ctrl Pts',(-90.9421739469738,44.3976534031992,82.2269238248473));
#38436=CARTESIAN_POINT('Ctrl Pts',(-90.9497795237996,44.3978625532565,78.6627969634214));
#38437=CARTESIAN_POINT('Ctrl Pts',(-91.4371495108539,43.6456431137721,75.1580571613055));
#38438=CARTESIAN_POINT('Ctrl Pts',(-92.,42.2636577765815,72.6550581100958));
#38439=CARTESIAN_POINT('Ctrl Pts',(-92.,41.,71.0942434347216));
#38440=CARTESIAN_POINT('Ctrl Pts',(-90.,39.24,72.0441908016846));
#38441=CARTESIAN_POINT('Ctrl Pts',(-90.,39.9925784091641,73.4385185783522));
#38442=CARTESIAN_POINT('Ctrl Pts',(-89.6247663405693,40.8156274544243,75.6745310640996));
#38443=CARTESIAN_POINT('Ctrl Pts',(-89.2998530158664,41.2636159206061,78.8054319539897));
#38444=CARTESIAN_POINT('Ctrl Pts',(-89.2947826313159,41.2634913601276,81.9893852835302));
#38445=CARTESIAN_POINT('Ctrl Pts',(-89.7999750759925,40.5929907863548,85.0924696714116));
#38446=CARTESIAN_POINT('Ctrl Pts',(-90.,39.616289204582,87.2586453099816));
#38447=CARTESIAN_POINT('Ctrl Pts',(-90.,39.24,87.9558091983154));
#38448=CARTESIAN_POINT('Origin',(-86.,41.,50.));
#38449=CARTESIAN_POINT('',(-92.,41.,50.));
#38450=CARTESIAN_POINT('',(-86.,47.,50.));
#38451=CARTESIAN_POINT('Origin',(-92.,24.5,80.));
#38452=CARTESIAN_POINT('',(-70.,24.5,96.75));
#38453=CARTESIAN_POINT('',(-92.,24.5,96.75));
#38454=CARTESIAN_POINT('Origin',(-70.,24.5,80.));
#38455=CARTESIAN_POINT('Origin',(-60.,15.,-125.));
#38456=CARTESIAN_POINT('',(-67.,15.,-125.));
#38457=CARTESIAN_POINT('Origin',(60.,15.,-125.));
#38458=CARTESIAN_POINT('',(53.,15.,-125.));
#38459=CARTESIAN_POINT('Origin',(-45.,24.5,114.));
#38460=CARTESIAN_POINT('',(-51.9,24.5,102.));
#38461=CARTESIAN_POINT('',(-51.9,24.5,114.));
#38462=CARTESIAN_POINT('Origin',(-45.,24.5,102.));
#38463=CARTESIAN_POINT('Origin',(-45.,24.5,102.));
#38464=CARTESIAN_POINT('Origin',(45.,24.5,114.));
#38465=CARTESIAN_POINT('',(38.1,24.5,102.));
#38466=CARTESIAN_POINT('',(38.1,24.5,114.));
#38467=CARTESIAN_POINT('Origin',(45.,24.5,102.));
#38468=CARTESIAN_POINT('Origin',(45.,24.5,102.));
#38469=CARTESIAN_POINT('Origin',(0.,24.5,110.));
#38470=CARTESIAN_POINT('',(-16.75,24.5,88.));
#38471=CARTESIAN_POINT('',(-16.75,24.5,110.));
#38472=CARTESIAN_POINT('Origin',(0.,24.5,88.));
#38473=CARTESIAN_POINT('Origin',(0.,24.5,88.));
#38474=CARTESIAN_POINT('Origin',(-70.,24.5,80.));
#38475=CARTESIAN_POINT('Origin',(-92.,41.,50.));
#38476=CARTESIAN_POINT('Origin',(70.,24.5,80.));
#38477=CARTESIAN_POINT('Origin',(92.,8.,50.));
#38478=CARTESIAN_POINT('',(92.,41.,50.));
#38479=CARTESIAN_POINT('',(92.,8.,50.));
#38480=CARTESIAN_POINT('',(92.,41.,50.));
#38481=CARTESIAN_POINT('Origin',(-41.0121933088198,48.,-41.0121933088198));
#38482=CARTESIAN_POINT('',(-46.0621933088198,28.,-41.0121933088198));
#38483=CARTESIAN_POINT('',(-46.0621933088198,48.,-41.0121933088198));
#38484=CARTESIAN_POINT('Origin',(-41.0121933088198,28.,-41.0121933088198));
#38485=CARTESIAN_POINT('Origin',(-41.0121933088198,28.,-41.0121933088198));
#38486=CARTESIAN_POINT('Origin',(-41.0121933088198,48.,41.0121933088198));
#38487=CARTESIAN_POINT('',(-46.0621933088198,28.,41.0121933088198));
#38488=CARTESIAN_POINT('',(-46.0621933088198,48.,41.0121933088198));
#38489=CARTESIAN_POINT('Origin',(-41.0121933088198,28.,41.0121933088198));
#38490=CARTESIAN_POINT('Origin',(-41.0121933088198,28.,41.0121933088198));
#38491=CARTESIAN_POINT('Origin',(41.0121933088198,48.,41.0121933088198));
#38492=CARTESIAN_POINT('',(35.9621933088198,28.,41.0121933088198));
#38493=CARTESIAN_POINT('',(35.9621933088198,48.,41.0121933088198));
#38494=CARTESIAN_POINT('Origin',(41.0121933088198,28.,41.0121933088198));
#38495=CARTESIAN_POINT('Origin',(41.0121933088198,28.,41.0121933088198));
#38496=CARTESIAN_POINT('Origin',(41.0121933088197,48.,-41.0121933088198));
#38497=CARTESIAN_POINT('',(35.9621933088197,28.,-41.0121933088198));
#38498=CARTESIAN_POINT('',(35.9621933088197,48.,-41.0121933088198));
#38499=CARTESIAN_POINT('Origin',(41.0121933088197,28.,-41.0121933088198));
#38500=CARTESIAN_POINT('Origin',(41.0121933088197,28.,-41.0121933088198));
#38501=CARTESIAN_POINT('Origin',(31.3800414539374,0.,-75.7581216659255));
#38502=CARTESIAN_POINT('',(26.3300414539374,20.,-75.7581216659255));
#38503=CARTESIAN_POINT('',(26.3300414539374,0.,-75.7581216659255));
#38504=CARTESIAN_POINT('Origin',(31.3800414539374,20.,-75.7581216659255));
#38505=CARTESIAN_POINT('Origin',(31.3800414539374,20.,-75.7581216659255));
#38506=CARTESIAN_POINT('Origin',(-75.7581216659255,0.,-31.3800414539373));
#38507=CARTESIAN_POINT('',(-80.8081216659255,20.,-31.3800414539373));
#38508=CARTESIAN_POINT('',(-80.8081216659255,0.,-31.3800414539373));
#38509=CARTESIAN_POINT('Origin',(-75.7581216659255,20.,-31.3800414539373));
#38510=CARTESIAN_POINT('Origin',(-75.7581216659255,20.,-31.3800414539373));
#38511=CARTESIAN_POINT('Origin',(-75.7581216659255,0.,31.3800414539374));
#38512=CARTESIAN_POINT('',(-80.8081216659255,20.,31.3800414539374));
#38513=CARTESIAN_POINT('',(-80.8081216659255,0.,31.3800414539374));
#38514=CARTESIAN_POINT('Origin',(-75.7581216659255,20.,31.3800414539374));
#38515=CARTESIAN_POINT('Origin',(-75.7581216659255,20.,31.3800414539374));
#38516=CARTESIAN_POINT('Origin',(31.3800414539374,0.,75.7581216659255));
#38517=CARTESIAN_POINT('',(26.3300414539374,20.,75.7581216659255));
#38518=CARTESIAN_POINT('',(26.3300414539374,0.,75.7581216659255));
#38519=CARTESIAN_POINT('Origin',(31.3800414539374,20.,75.7581216659255));
#38520=CARTESIAN_POINT('Origin',(31.3800414539374,20.,75.7581216659255));
#38521=CARTESIAN_POINT('Origin',(-31.3800414539374,0.,75.7581216659255));
#38522=CARTESIAN_POINT('',(-36.4300414539374,20.,75.7581216659255));
#38523=CARTESIAN_POINT('',(-36.4300414539374,0.,75.7581216659255));
#38524=CARTESIAN_POINT('Origin',(-31.3800414539374,20.,75.7581216659255));
#38525=CARTESIAN_POINT('Origin',(-31.3800414539374,20.,75.7581216659255));
#38526=CARTESIAN_POINT('Origin',(75.7581216659255,0.,31.3800414539374));
#38527=CARTESIAN_POINT('',(70.7081216659255,20.,31.3800414539374));
#38528=CARTESIAN_POINT('',(70.7081216659255,0.,31.3800414539374));
#38529=CARTESIAN_POINT('Origin',(75.7581216659255,20.,31.3800414539374));
#38530=CARTESIAN_POINT('Origin',(75.7581216659255,20.,31.3800414539374));
#38531=CARTESIAN_POINT('Origin',(-31.3800414539373,0.,-75.7581216659255));
#38532=CARTESIAN_POINT('',(-36.4300414539373,20.,-75.7581216659255));
#38533=CARTESIAN_POINT('',(-36.4300414539373,0.,-75.7581216659255));
#38534=CARTESIAN_POINT('Origin',(-31.3800414539373,20.,-75.7581216659255));
#38535=CARTESIAN_POINT('Origin',(-31.3800414539373,20.,-75.7581216659255));
#38536=CARTESIAN_POINT('Origin',(75.7581216659255,0.,-31.3800414539373));
#38537=CARTESIAN_POINT('',(70.7081216659255,20.,-31.3800414539373));
#38538=CARTESIAN_POINT('',(70.7081216659255,0.,-31.3800414539373));
#38539=CARTESIAN_POINT('Origin',(75.7581216659255,20.,-31.3800414539373));
#38540=CARTESIAN_POINT('Origin',(75.7581216659255,20.,-31.3800414539373));
#38541=CARTESIAN_POINT('Origin',(1.77635683940025E-14,9.,-4.70250832716619));
#38542=CARTESIAN_POINT('Origin',(0.,30.,13.));
#38543=CARTESIAN_POINT('',(-1.59204083889156E-15,30.,-13.));
#38544=CARTESIAN_POINT('Origin',(0.,30.,0.));
#38545=CARTESIAN_POINT('Origin',(0.,39.05,0.));
#38546=CARTESIAN_POINT('',(-1.59204083889156E-15,39.05,-13.));
#38547=CARTESIAN_POINT('Origin',(39.,30.5,110.));
#38548=CARTESIAN_POINT('',(39.,33.5,110.));
#38549=CARTESIAN_POINT('Origin',(51.,33.5,110.));
#38550=CARTESIAN_POINT('',(51.,33.5,110.));
#38551=CARTESIAN_POINT('Origin',(51.,30.5,110.));
#38552=CARTESIAN_POINT('',(54.,30.5,110.));
#38553=CARTESIAN_POINT('Origin',(54.,18.5,110.));
#38554=CARTESIAN_POINT('Origin',(-51.,30.5,110.));
#38555=CARTESIAN_POINT('',(-51.,33.5,110.));
#38556=CARTESIAN_POINT('Origin',(-39.,33.5,110.));
#38557=CARTESIAN_POINT('',(-39.,33.5,110.));
#38558=CARTESIAN_POINT('Origin',(-39.,30.5,110.));
#38559=CARTESIAN_POINT('',(-36.,30.5,110.));
#38560=CARTESIAN_POINT('Origin',(-36.,18.5,110.));
#38561=CARTESIAN_POINT('Origin',(-71.,-11.,-140.));
#38562=CARTESIAN_POINT('Origin',(39.,8.00000000000001,-125.));
#38563=CARTESIAN_POINT('',(39.,2.,-125.));
#38564=CARTESIAN_POINT('',(45.,8.,-125.));
#38565=CARTESIAN_POINT('Origin',(-39.,2.,-125.));
#38566=CARTESIAN_POINT('',(-39.,2.,-125.));
#38567=CARTESIAN_POINT('Origin',(-39.,8.00000000000001,-125.));
#38568=CARTESIAN_POINT('',(-45.,8.,-125.));
#38569=CARTESIAN_POINT('Origin',(-45.,36.,-125.));
#38570=CARTESIAN_POINT('',(-45.,36.,-125.));
#38571=CARTESIAN_POINT('Origin',(-39.,36.,-125.));
#38572=CARTESIAN_POINT('',(-39.,42.,-125.));
#38573=CARTESIAN_POINT('Origin',(39.,42.,-125.));
#38574=CARTESIAN_POINT('',(39.,42.,-125.));
#38575=CARTESIAN_POINT('Origin',(39.,36.,-125.));
#38576=CARTESIAN_POINT('',(45.,36.,-125.));
#38577=CARTESIAN_POINT('Origin',(45.,8.,-125.));
#38578=CARTESIAN_POINT('Origin',(0.,24.5,50.));
#38579=CARTESIAN_POINT('',(86.,47.,50.));
#38580=CARTESIAN_POINT('',(43.,47.,50.));
#38581=CARTESIAN_POINT('Origin',(86.,41.,50.));
#38582=CARTESIAN_POINT('Origin',(86.,47.,50.));
#38583=CARTESIAN_POINT('',(86.,47.,50.));
#38584=CARTESIAN_POINT('Origin',(86.,41.,50.));
#55695=UNCERTAINTY_MEASURE_WITH_UNIT(LENGTH_MEASURE(0.01),#55738,
'DISTANCE_ACCURACY_VALUE',
'Maximum model space distance between geometric entities at asserted c
onnectivities');
#55715=UNCERTAINTY_MEASURE_WITH_UNIT(LENGTH_MEASURE(0.01),#55738,
'DISTANCE_ACCURACY_VALUE',
'Maximum model space distance between geometric entities at asserted c
onnectivities');
#55717=(
GEOMETRIC_REPRESENTATION_CONTEXT(3)
GLOBAL_UNCERTAINTY_ASSIGNED_CONTEXT((#55695))
GLOBAL_UNIT_ASSIGNED_CONTEXT((#55738,#55740,#55741))
REPRESENTATION_CONTEXT('','3D')
);
#55737=(
GEOMETRIC_REPRESENTATION_CONTEXT(3)
GLOBAL_UNCERTAINTY_ASSIGNED_CONTEXT((#55715))
GLOBAL_UNIT_ASSIGNED_CONTEXT((#55738,#55740,#55741))
REPRESENTATION_CONTEXT('','3D')
);
#55738=(
LENGTH_UNIT()
NAMED_UNIT(*)
SI_UNIT(.MILLI.,.METRE.)
);
#55740=(
NAMED_UNIT(*)
PLANE_ANGLE_UNIT()
SI_UNIT($,.RADIAN.)
);
#55741=(
NAMED_UNIT(*)
SI_UNIT($,.STERADIAN.)
SOLID_ANGLE_UNIT()
);
#55743=SHAPE_DEFINITION_REPRESENTATION(#55764,#55821);
#55764=PRODUCT_DEFINITION_SHAPE('',$,#55843);
#55821=SHAPE_REPRESENTATION('',(#27463),#55717);
#55841=PRODUCT_DEFINITION_CONTEXT('part definition',#55906,'design');
#55843=PRODUCT_DEFINITION('2026-10-26-00-33-54-182','01_Pump_Casing',#55864,
#55841);
#55864=PRODUCT_DEFINITION_FORMATION('',$,#55909);
#55906=APPLICATION_CONTEXT(
'Core Data for Automotive Mechanical Design Process');
#55907=PRODUCT_CONTEXT('part definition',#55906,'mechanical');
#55909=PRODUCT('2026-10-26-00-33-54-182','01_Pump_Casing',$,(#55907));
#55999=COLOUR_RGB('Off White',0.89,0.88,0.83);
#56000=FILL_AREA_STYLE_COLOUR('',#55999);
#56001=FILL_AREA_STYLE('',(#56000));
#56002=SURFACE_STYLE_FILL_AREA(#56001);
#56003=SURFACE_SIDE_STYLE('',(#56002));
#56004=SURFACE_STYLE_USAGE(.BOTH.,#56003);
#56005=PRESENTATION_STYLE_ASSIGNMENT((#56004));
ENDSEC;
END-ISO-10303-21;
